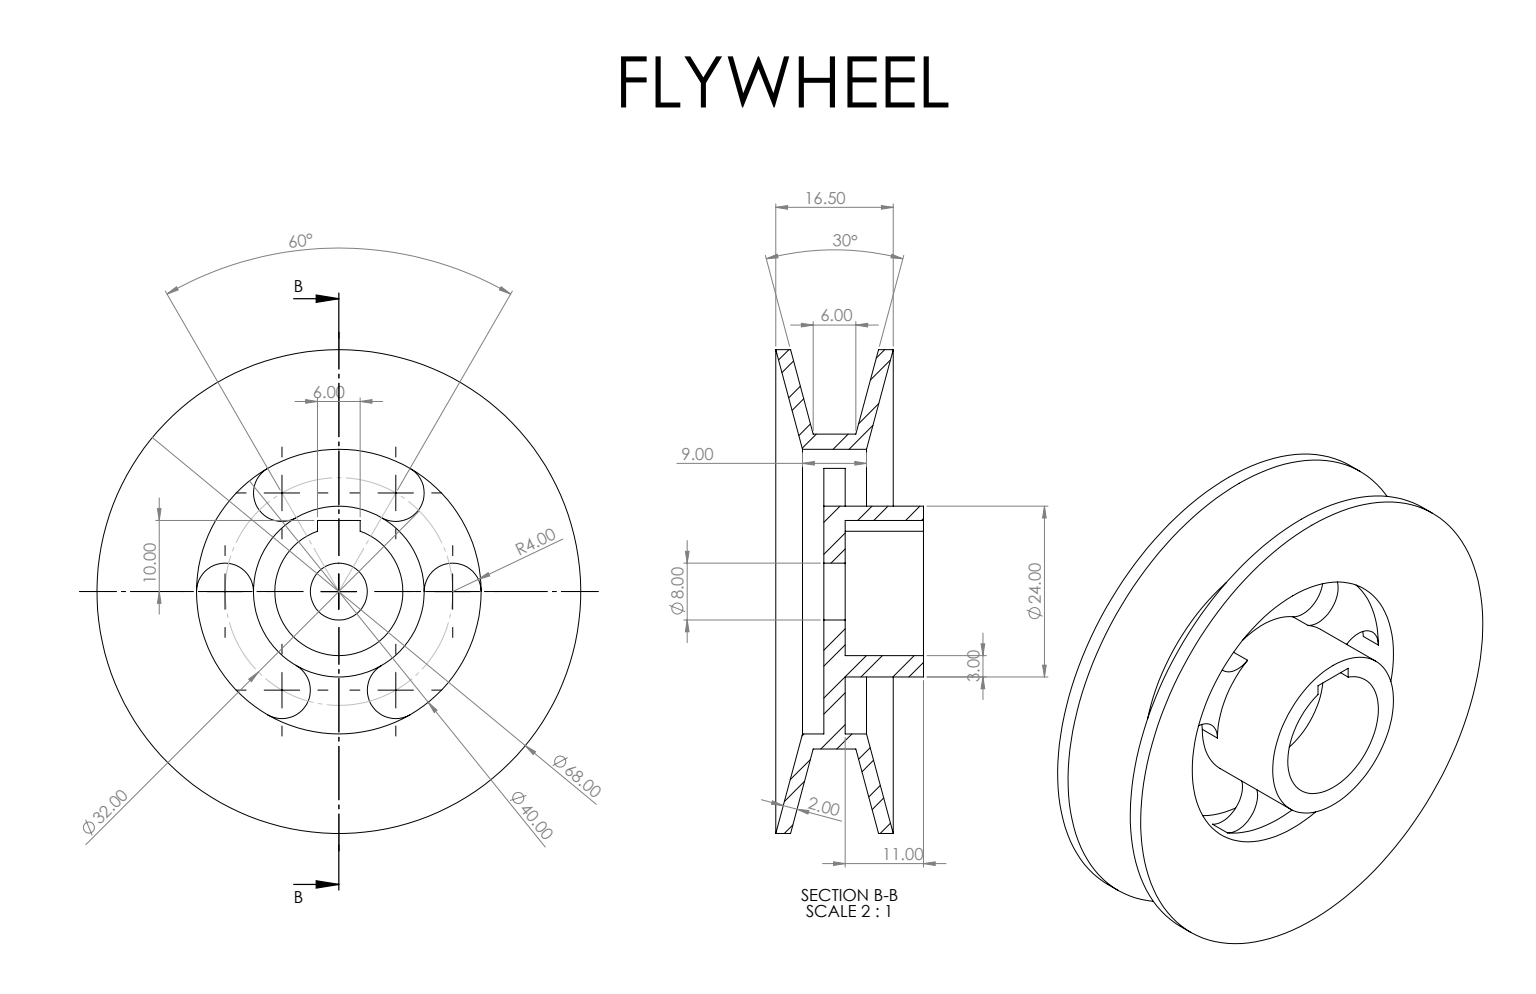
ISO-10303-21;
HEADER;
FILE_DESCRIPTION (('STEP AP214'),
    '1' );
FILE_NAME ('FLYWHEEL.step',
    '2026-10-24T00:51:42',
    ( '' ),
    ( '' ),
    'SwSTEP 2.0',
    'SolidWorks 2025',
    '' );
FILE_SCHEMA (( 'AUTOMOTIVE_DESIGN' ));
ENDSEC;

DATA;
#1=DIRECTION ( 'NONE',  ( 1.296372316667914327E-16, 1.000000000000000000, -0.000000000000000000 ) ) ;
#7=VERTEX_POINT ( 'NONE', #19816 ) ;
#14=LINE ( 'NONE', #10421, #6182 ) ;
#34=ORIENTED_EDGE ( 'NONE', *, *, #17370, .T. ) ;
#40=ORIENTED_EDGE ( 'NONE', *, *, #1892, .T. ) ;
#122=CARTESIAN_POINT ( 'NONE',  ( 4.000000000000007105, 28.19616000222403684, 4.898587196589412829E-16 ) ) ;
#157=DIRECTION ( 'NONE',  ( 0.000000000000000000, 0.000000000000000000, 1.000000000000000000 ) ) ;
#180=( LENGTH_UNIT ( ) NAMED_UNIT ( * ) SI_UNIT ( .MILLI., .METRE. ) );
#212=EDGE_LOOP ( 'NONE', ( #4099, #12246, #12145, #6281 ) ) ;
#220=AXIS2_PLACEMENT_3D ( 'NONE', #14083, #12166, #15923 ) ;
#229=ORIENTED_EDGE ( 'NONE', *, *, #280, .F. ) ;
#235=CARTESIAN_POINT ( 'NONE',  ( 34.00000000000000000, -8.251288694035739724, 4.163799117101000559E-15 ) ) ;
#250=( NAMED_UNIT ( * ) SI_UNIT ( $, .STERADIAN. ) SOLID_ANGLE_UNIT ( ) );
#252=ORIENTED_EDGE ( 'NONE', *, *, #20268, .F. ) ;
#272=VECTOR ( 'NONE', #9542, 1000.000000000000000 ) ;
#273=VECTOR ( 'NONE', #6613, 1000.000000000000000 ) ;
#280=EDGE_CURVE ( 'NONE', #4403, #3845, #2016, .T. ) ;
#286=DIRECTION ( 'NONE',  ( 1.000000000000000000, -1.084202172485504927E-16, 0.000000000000000000 ) ) ;
#298=DIRECTION ( 'NONE',  ( -1.000000000000000000, 0.000000000000000000, 0.000000000000000000 ) ) ;
#301=AXIS2_PLACEMENT_3D ( 'NONE', #19951, #21671, #11581 ) ;
#316=AXIS2_PLACEMENT_3D ( 'NONE', #15240, #12961, #19969 ) ;
#342=DIRECTION ( 'NONE',  ( -1.000000000000000000, 0.000000000000000000, 0.000000000000000000 ) ) ;
#354=DIRECTION ( 'NONE',  ( 1.296372316667914327E-16, 1.000000000000000000, -0.000000000000000000 ) ) ;
#379=CARTESIAN_POINT ( 'NONE',  ( -13.85640646055084702, -1.500000000000011768, 7.999999999999705125 ) ) ;
#395=EDGE_LOOP ( 'NONE', ( #16035, #6473, #11617, #1674 ) ) ;
#397=EDGE_CURVE ( 'NONE', #22398, #3259, #6731, .T. ) ;
#414=CIRCLE ( 'NONE', #13204, 4.000000000000000000 ) ;
#421=PLANE ( 'NONE',  #17700 ) ;
#422=CARTESIAN_POINT ( 'NONE',  ( 34.00000000000000000, 8.251288694035739724, 4.163799117100999770E-15 ) ) ;
#432=ORIENTED_EDGE ( 'NONE', *, *, #17613, .T. ) ;
#435=DIRECTION ( 'NONE',  ( -1.000000000000000000, 1.371829164384562918E-16, 0.000000000000000000 ) ) ;
#439=FACE_OUTER_BOUND ( 'NONE', #4503, .T. ) ;
#457=DIRECTION ( 'NONE',  ( 1.296372316667914327E-16, 1.000000000000000000, -0.000000000000000000 ) ) ;
#480=LINE ( 'NONE', #7251, #20898 ) ;
#494=CARTESIAN_POINT ( 'NONE',  ( 3.849727973822421485E-15, 1.499999999999994449, 0.000000000000000000 ) ) ;
#501=EDGE_CURVE ( 'NONE', #11241, #8065, #19539, .T. ) ;
#512=VECTOR ( 'NONE', #9586, 1000.000000000000000 ) ;
#517=DIRECTION ( 'NONE',  ( 1.296372316667914327E-16, 1.000000000000000000, -0.000000000000000000 ) ) ;
#518=VECTOR ( 'NONE', #17062, 1000.000000000000000 ) ;
#522=DIRECTION ( 'NONE',  ( 1.296372316667914327E-16, 1.000000000000000000, -0.000000000000000000 ) ) ;
#549=EDGE_CURVE ( 'NONE', #21392, #4403, #13704, .T. ) ;
#562=AXIS2_PLACEMENT_3D ( 'NONE', #8192, #22408, #11628 ) ;
#569=CARTESIAN_POINT ( 'NONE',  ( -13.85640646055084702, -1.500000000000011768, 11.99999999999970335 ) ) ;
#570=CIRCLE ( 'NONE', #3154, 19.99999999999999289 ) ;
#577=AXIS2_PLACEMENT_3D ( 'NONE', #19256, #1, #8819 ) ;
#598=( LENGTH_UNIT ( ) NAMED_UNIT ( * ) SI_UNIT ( .MILLI., .METRE. ) );
#610=DIRECTION ( 'NONE',  ( 1.000000000000000000, -1.301042606982605814E-16, 0.000000000000000000 ) ) ;
#621=EDGE_CURVE ( 'NONE', #21949, #5947, #10354, .T. ) ;
#626=VERTEX_POINT ( 'NONE', #3731 ) ;
#627=ORIENTED_EDGE ( 'NONE', *, *, #19282, .F. ) ;
#644=CARTESIAN_POINT ( 'NONE',  ( -22.12933039895921183, -2.999999999999992895, 0.000000000000000000 ) ) ;
#651=VERTEX_POINT ( 'NONE', #17468 ) ;
#656=AXIS2_PLACEMENT_3D ( 'NONE', #1334, #18751, #13229 ) ;
#659=CARTESIAN_POINT ( 'NONE',  ( 4.000000000000003553, -1.500000000000015099, 0.000000000000000000 ) ) ;
#669=CIRCLE ( 'NONE', #11643, 22.12933039895921539 ) ;
#676=ORIENTED_EDGE ( 'NONE', *, *, #4878, .T. ) ;
#694=DIRECTION ( 'NONE',  ( 1.296372316667914327E-16, 1.000000000000000000, -0.000000000000000000 ) ) ;
#780=CARTESIAN_POINT ( 'NONE',  ( -17.32050807568873196, -1.500000000000011768, 9.999999999999772626 ) ) ;
#782=FACE_OUTER_BOUND ( 'NONE', #19177, .T. ) ;
#793=DIRECTION ( 'NONE',  ( 1.296372316667914327E-16, 1.000000000000000000, -0.000000000000000000 ) ) ;
#881=FACE_BOUND ( 'NONE', #13282, .T. ) ;
#888=CARTESIAN_POINT ( 'NONE',  ( 34.00000000000000711, 28.19616000222403329, 4.163799117101000559E-15 ) ) ;
#902=CARTESIAN_POINT ( 'NONE',  ( 13.85640646055130709, -1.500000000000015099, -4.000000000000099476 ) ) ;
#918=DIRECTION ( 'NONE',  ( -1.000000000000000000, 0.000000000000000000, 0.000000000000000000 ) ) ;
#925=CYLINDRICAL_SURFACE ( 'NONE', #17707, 4.000000000000000000 ) ;
#931=CIRCLE ( 'NONE', #17391, 9.000000000000000000 ) ;
#946=ORIENTED_EDGE ( 'NONE', *, *, #15805, .F. ) ;
#970=VECTOR ( 'NONE', #5351, 1000.000000000000000 ) ;
#988=CARTESIAN_POINT ( 'NONE',  ( 1.734786545154649763E-13, 1.500000000000004885, -16.00000000000029488 ) ) ;
#1012=EDGE_CURVE ( 'NONE', #17260, #11580, #15474, .T. ) ;
#1095=ORIENTED_EDGE ( 'NONE', *, *, #6767, .T. ) ;
#1099=ORIENTED_EDGE ( 'NONE', *, *, #9484, .F. ) ;
#1215=VECTOR ( 'NONE', #22012, 1000.000000000000000 ) ;
#1276=CARTESIAN_POINT ( 'NONE',  ( -19.99999999999998934, 4.500000000000009770, 0.000000000000000000 ) ) ;
#1326=AXIS2_PLACEMENT_3D ( 'NONE', #12628, #3503, #21247 ) ;
#1334=CARTESIAN_POINT ( 'NONE',  ( 7.310544252644470693E-15, 28.19616000222403684, 0.000000000000000000 ) ) ;
#1341=CARTESIAN_POINT ( 'NONE',  ( -10.00000000000000000, 1.499999999999997780, 3.000000000000000000 ) ) ;
#1373=VECTOR ( 'NONE', #12449, 1000.000000000000000 ) ;
#1375=ORIENTED_EDGE ( 'NONE', *, *, #8971, .T. ) ;
#1384=CIRCLE ( 'NONE', #21527, 3.999999999999996447 ) ;
#1398=DIRECTION ( 'NONE',  ( 0.000000000000000000, 0.000000000000000000, 1.000000000000000000 ) ) ;
#1399=APPLICATION_CONTEXT ( 'automotive_design' ) ;
#1406=ORIENTED_EDGE ( 'NONE', *, *, #8971, .F. ) ;
#1427=ORIENTED_EDGE ( 'NONE', *, *, #4182, .T. ) ;
#1436=CARTESIAN_POINT ( 'NONE',  ( 20.00000000000000000, 28.19616000222403329, 2.449293598294705724E-15 ) ) ;
#1444=( GEOMETRIC_REPRESENTATION_CONTEXT ( 3 ) GLOBAL_UNCERTAINTY_ASSIGNED_CONTEXT ( ( #13302 ) ) GLOBAL_UNIT_ASSIGNED_CONTEXT ( ( #598, #9306, #250 ) ) REPRESENTATION_CONTEXT ( 'NONE', 'WORKASPACE' ) );
#1469=DIRECTION ( 'NONE',  ( 1.296372316667914327E-16, 1.000000000000000000, -0.000000000000000000 ) ) ;
#1505=EDGE_CURVE ( 'NONE', #15515, #14562, #11061, .T. ) ;
#1506=FACE_BOUND ( 'NONE', #395, .T. ) ;
#1516=ORIENTED_EDGE ( 'NONE', *, *, #3101, .T. ) ;
#1526=DIRECTION ( 'NONE',  ( -1.000000000000000000, 1.927470528863119049E-16, 0.000000000000000000 ) ) ;
#1552=ORIENTED_EDGE ( 'NONE', *, *, #2402, .F. ) ;
#1570=ORIENTED_EDGE ( 'NONE', *, *, #10768, .F. ) ;
#1595=FACE_OUTER_BOUND ( 'NONE', #17651, .T. ) ;
#1624=CARTESIAN_POINT ( 'NONE',  ( 3.849727973822421485E-15, 1.499999999999997780, 0.000000000000000000 ) ) ;
#1638=DIRECTION ( 'NONE',  ( -1.000000000000000000, 1.734723475976807834E-16, 0.000000000000000000 ) ) ;
#1642=EDGE_CURVE ( 'NONE', #7946, #651, #17286, .T. ) ;
#1648=CARTESIAN_POINT ( 'NONE',  ( 0.000000000000000000, 0.000000000000000000, 0.000000000000000000 ) ) ;
#1649=ORIENTED_EDGE ( 'NONE', *, *, #7636, .F. ) ;
#1650=DIRECTION ( 'NONE',  ( 1.296372316667914327E-16, 1.000000000000000000, -0.000000000000000000 ) ) ;
#1658=ORIENTED_EDGE ( 'NONE', *, *, #14495, .T. ) ;
#1661=EDGE_LOOP ( 'NONE', ( #6020, #16109, #16262, #15546 ) ) ;
#1663=AXIS2_PLACEMENT_3D ( 'NONE', #9499, #12798, #435 ) ;
#1664=CARTESIAN_POINT ( 'NONE',  ( -34.00000000000000000, -6.180736333215561373, 4.163799117101000559E-15 ) ) ;
#1674=ORIENTED_EDGE ( 'NONE', *, *, #1642, .T. ) ;
#1682=VECTOR ( 'NONE', #1745, 1000.000000000000000 ) ;
#1684=AXIS2_PLACEMENT_3D ( 'NONE', #17713, #14492, #2138 ) ;
#1696=AXIS2_PLACEMENT_3D ( 'NONE', #22355, #2878, #22124 ) ;
#1713=FACE_OUTER_BOUND ( 'NONE', #5783, .T. ) ;
#1735=CARTESIAN_POINT ( 'NONE',  ( 22.12933039895921894, 3.000000000000003109, 3.436930240568481542E-15 ) ) ;
#1745=DIRECTION ( 'NONE',  ( 1.296372316667914327E-16, 1.000000000000000000, -0.000000000000000000 ) ) ;
#1747=ORIENTED_EDGE ( 'NONE', *, *, #6797, .T. ) ;
#1756=FACE_OUTER_BOUND ( 'NONE', #13620, .T. ) ;
#1775=ORIENTED_EDGE ( 'NONE', *, *, #13470, .T. ) ;
#1788=CARTESIAN_POINT ( 'NONE',  ( -2.467804172277818612E-14, 1.500000000000002887, 11.99999999999966960 ) ) ;
#1797=DIRECTION ( 'NONE',  ( 1.296372316667914327E-16, 1.000000000000000000, -0.000000000000000000 ) ) ;
#1808=CARTESIAN_POINT ( 'NONE',  ( -22.12933039895921183, 3.000000000000009326, 0.000000000000000000 ) ) ;
#1892=EDGE_CURVE ( 'NONE', #8190, #7904, #20239, .T. ) ;
#1895=AXIS2_PLACEMENT_3D ( 'NONE', #17411, #3457, #6656 ) ;
#1898=ORIENTED_EDGE ( 'NONE', *, *, #11064, .F. ) ;
#1918=ORIENTED_EDGE ( 'NONE', *, *, #10579, .T. ) ;
#1985=VERTEX_POINT ( 'NONE', #12497 ) ;
#2016=CIRCLE ( 'NONE', #19183, 19.99999999999999289 ) ;
#2024=CARTESIAN_POINT ( 'NONE',  ( -10.39230484541309174, -1.500000000000011768, 5.999999999999708677 ) ) ;
#2027=ORIENTED_EDGE ( 'NONE', *, *, #12241, .F. ) ;
#2044=ORIENTED_EDGE ( 'NONE', *, *, #10253, .T. ) ;
#2061=DIRECTION ( 'NONE',  ( 0.000000000000000000, 0.000000000000000000, 1.000000000000000000 ) ) ;
#2132=DIRECTION ( 'NONE',  ( -0.000000000000000000, 1.000000000000000000, -0.000000000000000000 ) ) ;
#2137=CYLINDRICAL_SURFACE ( 'NONE', #9464, 8.999999999999998224 ) ;
#2138=DIRECTION ( 'NONE',  ( -1.000000000000000000, 1.084202172485504434E-16, 0.000000000000000000 ) ) ;
#2160=CARTESIAN_POINT ( 'NONE',  ( -10.00000000000000000, 1.499999999999997780, 3.000000000000000000 ) ) ;
#2189=ADVANCED_FACE ( 'NONE', ( #6551 ), #19147, .T. ) ;
#2257=EDGE_LOOP ( 'NONE', ( #1570, #15899 ) ) ;
#2264=DIRECTION ( 'NONE',  ( 1.296372316667914327E-16, 1.000000000000000000, -0.000000000000000000 ) ) ;
#2296=EDGE_CURVE ( 'NONE', #10675, #16483, #414, .T. ) ;
#2304=VERTEX_POINT ( 'NONE', #569 ) ;
#2307=DIRECTION ( 'NONE',  ( 1.296372316667914327E-16, 1.000000000000000000, -0.000000000000000000 ) ) ;
#2362=DIRECTION ( 'NONE',  ( -1.000000000000000000, 1.371829164384562918E-16, 0.000000000000000000 ) ) ;
#2369=AXIS2_PLACEMENT_3D ( 'NONE', #22218, #1469, #20718 ) ;
#2376=CARTESIAN_POINT ( 'NONE',  ( 9.000000000000005329, 12.49999999999999467, 0.000000000000000000 ) ) ;
#2377=CLOSED_SHELL ( 'NONE', ( #15840, #2588, #18828, #3195, #14125, #19318, #13827, #6682, #21945, #10747, #17338, #14273, #22672, #14010, #8312, #12983, #9918, #6676, #7246, #21227, #12866, #3900, #16028, #2189, #18705, #11982, #13364, #12111, #21806, #17586, #11435, #17237, #8288, #21448, #10491, #16012, #20701, #9854 ) ) ;
#2380=EDGE_CURVE ( 'NONE', #8634, #18457, #2887, .T. ) ;
#2402=EDGE_CURVE ( 'NONE', #12588, #11670, #15669, .T. ) ;
#2415=ORIENTED_EDGE ( 'NONE', *, *, #1505, .T. ) ;
#2424=CARTESIAN_POINT ( 'NONE',  ( 12.00000000000000355, 1.499999999999996447, 1.469576158976823947E-15 ) ) ;
#2449=ORIENTED_EDGE ( 'NONE', *, *, #5012, .F. ) ;
#2475=CYLINDRICAL_SURFACE ( 'NONE', #21721, 12.00000000000000000 ) ;
#2497=CARTESIAN_POINT ( 'NONE',  ( 4.044183821322609990E-15, 3.000000000000006217, 0.000000000000000000 ) ) ;
#2507=DIRECTION ( 'NONE',  ( -1.000000000000000000, 1.567804759296643123E-16, 0.000000000000000000 ) ) ;
#2511=VECTOR ( 'NONE', #20802, 1000.000000000000000 ) ;
#2514=DIRECTION ( 'NONE',  ( -1.000000000000000000, 0.000000000000000000, -0.000000000000000000 ) ) ;
#2530=ORIENTED_EDGE ( 'NONE', *, *, #6684, .T. ) ;
#2575=STYLED_ITEM('',(#22748),#18432);
#2588=ADVANCED_FACE ( 'NONE', ( #9466 ), #19884, .F. ) ;
#2610=FACE_BOUND ( 'NONE', #18350, .T. ) ;
#2630=EDGE_CURVE ( 'NONE', #3259, #22398, #13450, .T. ) ;
#2640=CARTESIAN_POINT ( 'NONE',  ( -13.85640646055084702, -25.00000000000000000, 7.999999999999705125 ) ) ;
#2659=EDGE_CURVE ( 'NONE', #6902, #13173, #9095, .T. ) ;
#2683=DIRECTION ( 'NONE',  ( -1.000000000000000000, 1.530638361156006245E-16, 0.000000000000000000 ) ) ;
#2739=CARTESIAN_POINT ( 'NONE',  ( -33.99999999999998579, 8.251288694035750382, 0.000000000000000000 ) ) ;
#2745=EDGE_CURVE ( 'NONE', #8634, #14562, #13436, .T. ) ;
#2747=CARTESIAN_POINT ( 'NONE',  ( -4.359932693009644117E-14, -1.500000000000015987, 19.99999999999999289 ) ) ;
#2803=AXIS2_PLACEMENT_3D ( 'NONE', #18547, #21883, #16594 ) ;
#2812=ORIENTED_EDGE ( 'NONE', *, *, #21989, .F. ) ;
#2821=DIRECTION ( 'NONE',  ( 1.296372316667914327E-16, 1.000000000000000000, -0.000000000000000000 ) ) ;
#2829=EDGE_CURVE ( 'NONE', #18519, #22196, #7986, .T. ) ;
#2831=ORIENTED_EDGE ( 'NONE', *, *, #18843, .T. ) ;
#2847=AXIS2_PLACEMENT_3D ( 'NONE', #3112, #11479, #18699 ) ;
#2871=DIRECTION ( 'NONE',  ( 1.296372316667914327E-16, 1.000000000000000000, -0.000000000000000000 ) ) ;
#2878=DIRECTION ( 'NONE',  ( 1.296372316667914327E-16, 1.000000000000000000, -0.000000000000000000 ) ) ;
#2887=CIRCLE ( 'NONE', #3984, 22.12933039895921539 ) ;
#2903=FACE_OUTER_BOUND ( 'NONE', #3500, .T. ) ;
#2924=AXIS2_PLACEMENT_3D ( 'NONE', #12514, #12753, #3836 ) ;
#2961=LINE ( 'NONE', #7881, #22187 ) ;
#3024=CYLINDRICAL_SURFACE ( 'NONE', #17665, 34.00000000000000000 ) ;
#3101=EDGE_CURVE ( 'NONE', #5844, #9303, #19375, .T. ) ;
#3103=ORIENTED_EDGE ( 'NONE', *, *, #397, .F. ) ;
#3112=CARTESIAN_POINT ( 'NONE',  ( 3.071904583821672593E-15, -4.500000000000010658, 0.000000000000000000 ) ) ;
#3115=CARTESIAN_POINT ( 'NONE',  ( -22.12933039895921183, 3.000000000000009326, 0.000000000000000000 ) ) ;
#3154=AXIS2_PLACEMENT_3D ( 'NONE', #8531, #8978, #7380 ) ;
#3161=AXIS2_PLACEMENT_3D ( 'NONE', #22565, #17265, #13584 ) ;
#3163=EDGE_CURVE ( 'NONE', #17046, #6470, #17144, .T. ) ;
#3174=AXIS2_PLACEMENT_3D ( 'NONE', #3756, #12999, #4437 ) ;
#3195=ADVANCED_FACE ( 'NONE', ( #2903 ), #9110, .F. ) ;
#3233=FACE_OUTER_BOUND ( 'NONE', #11673, .T. ) ;
#3254=CARTESIAN_POINT ( 'NONE',  ( 5.275737522157127195E-15, 12.49999999999999645, 0.000000000000000000 ) ) ;
#3259=VERTEX_POINT ( 'NONE', #3115 ) ;
#3291=ORIENTED_EDGE ( 'NONE', *, *, #10893, .F. ) ;
#3292=CARTESIAN_POINT ( 'NONE',  ( 2.854018578421813982E-15, -6.180736333215565814, 0.000000000000000000 ) ) ;
#3303=LINE ( 'NONE', #1341, #273 ) ;
#3314=CIRCLE ( 'NONE', #14983, 19.99999999999999289 ) ;
#3317=EDGE_CURVE ( 'NONE', #4351, #21949, #14, .T. ) ;
#3334=CARTESIAN_POINT ( 'NONE',  ( 12.00000000000000711, 28.19616000222403684, 1.469576158976823947E-15 ) ) ;
#3355=CARTESIAN_POINT ( 'NONE',  ( -10.39230484541300825, -1.500000000000011768, -6.000000000000442313 ) ) ;
#3362=ORIENTED_EDGE ( 'NONE', *, *, #549, .F. ) ;
#3363=CARTESIAN_POINT ( 'NONE',  ( 6.383438919230843859E-14, -25.00000000000000000, -20.00000000000029488 ) ) ;
#3367=CARTESIAN_POINT ( 'NONE',  ( 7.310544252644470693E-15, 28.19616000222403684, 0.000000000000000000 ) ) ;
#3401=EDGE_CURVE ( 'NONE', #7, #1985, #4720, .T. ) ;
#3402=CARTESIAN_POINT ( 'NONE',  ( -8.485281374238564212, 12.49999999999999822, -3.000000000000000000 ) ) ;
#3407=ORIENTED_EDGE ( 'NONE', *, *, #12251, .F. ) ;
#3446=PLANE ( 'NONE',  #9367 ) ;
#3457=DIRECTION ( 'NONE',  ( 1.296372316667914327E-16, 1.000000000000000000, -0.000000000000000000 ) ) ;
#3467=DIRECTION ( 'NONE',  ( 1.296372316667914327E-16, 1.000000000000000000, -0.000000000000000000 ) ) ;
#3475=ORIENTED_EDGE ( 'NONE', *, *, #2296, .F. ) ;
#3500=EDGE_LOOP ( 'NONE', ( #2831, #8629, #10943, #13779 ) ) ;
#3503=DIRECTION ( 'NONE',  ( 1.296372316667914327E-16, 1.000000000000000000, -0.000000000000000000 ) ) ;
#3511=EDGE_LOOP ( 'NONE', ( #18181, #22428, #18359, #11116 ) ) ;
#3519=DIRECTION ( 'NONE',  ( -1.000000000000000000, 1.264902534566421922E-16, 0.000000000000000000 ) ) ;
#3541=ORIENTED_EDGE ( 'NONE', *, *, #7207, .F. ) ;
#3550=CARTESIAN_POINT ( 'NONE',  ( 7.310544252644470693E-15, 28.19616000222403684, 0.000000000000000000 ) ) ;
#3555=AXIS2_PLACEMENT_3D ( 'NONE', #21855, #6153, #16567 ) ;
#3565=EDGE_CURVE ( 'NONE', #20227, #17027, #10702, .T. ) ;
#3573=VECTOR ( 'NONE', #18015, 1000.000000000000000 ) ;
#3583=LINE ( 'NONE', #7883, #7896 ) ;
#3612=DIRECTION ( 'NONE',  ( 1.296372316667914327E-16, 1.000000000000000000, -0.000000000000000000 ) ) ;
#3616=ORIENTED_EDGE ( 'NONE', *, *, #3163, .F. ) ;
#3635=VERTEX_POINT ( 'NONE', #11450 ) ;
#3669=ORIENTED_EDGE ( 'NONE', *, *, #10893, .T. ) ;
#3671=DIRECTION ( 'NONE',  ( 1.296372316667914327E-16, 1.000000000000000000, -0.000000000000000000 ) ) ;
#3731=CARTESIAN_POINT ( 'NONE',  ( 13.85640646055130709, 1.500000000000004885, -4.000000000000099476 ) ) ;
#3756=CARTESIAN_POINT ( 'NONE',  ( 3.849727973822421485E-15, 1.499999999999997780, 0.000000000000000000 ) ) ;
#3771=DIRECTION ( 'NONE',  ( 0.9659258262890680902, -0.2588190451025210170, 0.000000000000000000 ) ) ;
#3778=CARTESIAN_POINT ( 'NONE',  ( 12.00000000000000355, 1.500000000000003553, 0.000000000000000000 ) ) ;
#3780=VECTOR ( 'NONE', #5970, 1000.000000000000000 ) ;
#3825=CARTESIAN_POINT ( 'NONE',  ( 10.39230484541348432, 1.500000000000003109, -6.000000000000073719 ) ) ;
#3827=LINE ( 'NONE', #3942, #3573 ) ;
#3836=DIRECTION ( 'NONE',  ( -1.000000000000000000, 1.301042606982605814E-16, 0.000000000000000000 ) ) ;
#3845=VERTEX_POINT ( 'NONE', #4000 ) ;
#3847=EDGE_LOOP ( 'NONE', ( #20703, #21022, #16887, #11706 ) ) ;
#3855=CIRCLE ( 'NONE', #9702, 11.99999999999985256 ) ;
#3859=DIRECTION ( 'NONE',  ( -1.000000000000000000, 1.084202172485504927E-16, 0.000000000000000000 ) ) ;
#3889=ORIENTED_EDGE ( 'NONE', *, *, #2659, .F. ) ;
#3891=CARTESIAN_POINT ( 'NONE',  ( -10.00000000000000000, -4.824555320336763486, -3.000000000000000000 ) ) ;
#3900=ADVANCED_FACE ( 'NONE', ( #21293 ), #8809, .T. ) ;
#3919=DIRECTION ( 'NONE',  ( -1.296372316667914327E-16, -1.000000000000000000, 0.000000000000000000 ) ) ;
#3942=CARTESIAN_POINT ( 'NONE',  ( -8.485281374238560659, 28.19616000222403684, -3.000000000000000000 ) ) ;
#3964=ORIENTED_EDGE ( 'NONE', *, *, #10073, .F. ) ;
#3984=AXIS2_PLACEMENT_3D ( 'NONE', #12211, #19213, #19095 ) ;
#3994=DIRECTION ( 'NONE',  ( -1.000000000000000000, 1.371829164384562918E-16, 0.000000000000000000 ) ) ;
#4000=CARTESIAN_POINT ( 'NONE',  ( 17.32050807568880657, -1.500000000000015987, -9.999999999999934275 ) ) ;
#4004=CARTESIAN_POINT ( 'NONE',  ( 20.00000000000000000, 28.19616000222403329, 2.449293598294705724E-15 ) ) ;
#4014=CARTESIAN_POINT ( 'NONE',  ( -9.999999999999998224, 12.49999999999999822, 3.000000000000000000 ) ) ;
#4044=VERTEX_POINT ( 'NONE', #4106 ) ;
#4053=CARTESIAN_POINT ( 'NONE',  ( -8.485281374238564212, 1.499999999999997558, -3.000000000000000000 ) ) ;
#4099=ORIENTED_EDGE ( 'NONE', *, *, #21744, .F. ) ;
#4106=CARTESIAN_POINT ( 'NONE',  ( -8.485281374238564212, 12.49999999999999822, 3.000000000000000000 ) ) ;
#4147=DIRECTION ( 'NONE',  ( 1.296372316667914327E-16, 1.000000000000000000, -0.000000000000000000 ) ) ;
#4182=EDGE_CURVE ( 'NONE', #5980, #4044, #8889, .T. ) ;
#4192=CONICAL_SURFACE ( 'NONE', #6735, 22.12933039895921539, 1.308996938995746095 ) ;
#4230=LINE ( 'NONE', #2739, #17492 ) ;
#4231=AXIS2_PLACEMENT_3D ( 'NONE', #7568, #457, #918 ) ;
#4299=EDGE_CURVE ( 'NONE', #14562, #15515, #14533, .T. ) ;
#4332=CARTESIAN_POINT ( 'NONE',  ( 0.000000000000000000, -25.00000000000000000, 11.99999999999985256 ) ) ;
#4351=VERTEX_POINT ( 'NONE', #4053 ) ;
#4354=DIRECTION ( 'NONE',  ( 1.296372316667914327E-16, 1.000000000000000000, -0.000000000000000000 ) ) ;
#4380=PRODUCT_DEFINITION_SHAPE ( 'NONE', 'NONE',  #17947 ) ;
#4392=CARTESIAN_POINT ( 'NONE',  ( 3.071904583821672593E-15, -4.500000000000010658, 0.000000000000000000 ) ) ;
#4403=VERTEX_POINT ( 'NONE', #18462 ) ;
#4407=UNCERTAINTY_MEASURE_WITH_UNIT (LENGTH_MEASURE( 1.000000000000000082E-05 ), #180, 'distance_accuracy_value', 'NONE');
#4437=DIRECTION ( 'NONE',  ( -1.000000000000000000, 1.264902534566421922E-16, 0.000000000000000000 ) ) ;
#4446=DIRECTION ( 'NONE',  ( -1.000000000000000000, 1.084202172485504434E-16, 0.000000000000000000 ) ) ;
#4475=DIRECTION ( 'NONE',  ( -0.000000000000000000, 1.000000000000000000, -0.000000000000000000 ) ) ;
#4503=EDGE_LOOP ( 'NONE', ( #16138, #13930, #14702, #3407 ) ) ;
#4540=ORIENTED_EDGE ( 'NONE', *, *, #11064, .T. ) ;
#4548=AXIS2_PLACEMENT_3D ( 'NONE', #988, #13222, #16801 ) ;
#4580=EDGE_CURVE ( 'NONE', #5486, #5841, #20871, .T. ) ;
#4592=EDGE_CURVE ( 'NONE', #17027, #20227, #5906, .T. ) ;
#4599=CIRCLE ( 'NONE', #562, 3.999999999999996447 ) ;
#4614=CARTESIAN_POINT ( 'NONE',  ( 0.000000000000000000, 1.500000000000015099, 19.99999999999999645 ) ) ;
#4622=EDGE_CURVE ( 'NONE', #8683, #5161, #12467, .T. ) ;
#4633=AXIS2_PLACEMENT_3D ( 'NONE', #13899, #15504, #17117 ) ;
#4654=CONICAL_SURFACE ( 'NONE', #7559, 19.99999999999999289, 1.308996938995746984 ) ;
#4665=EDGE_LOOP ( 'NONE', ( #8035, #2027, #11749, #12833 ) ) ;
#4676=ORIENTED_EDGE ( 'NONE', *, *, #3401, .F. ) ;
#4696=EDGE_LOOP ( 'NONE', ( #14995, #20897, #432, #14474 ) ) ;
#4704=AXIS2_PLACEMENT_3D ( 'NONE', #8446, #5352, #8891 ) ;
#4717=ORIENTED_EDGE ( 'NONE', *, *, #621, .F. ) ;
#4720=CIRCLE ( 'NONE', #18620, 33.99999999999999289 ) ;
#4741=EDGE_LOOP ( 'NONE', ( #1552, #1747, #1516, #16833, #19996 ) ) ;
#4798=FACE_OUTER_BOUND ( 'NONE', #17306, .T. ) ;
#4799=FACE_BOUND ( 'NONE', #2257, .T. ) ;
#4812=CARTESIAN_POINT ( 'NONE',  ( -13.85640646055084702, 1.500000000000008216, 11.99999999999970335 ) ) ;
#4831=ORIENTED_EDGE ( 'NONE', *, *, #10006, .T. ) ;
#4878=EDGE_CURVE ( 'NONE', #18308, #22383, #7725, .T. ) ;
#4914=VECTOR ( 'NONE', #6786, 1000.000000000000000 ) ;
#4943=CARTESIAN_POINT ( 'NONE',  ( -13.85640646055073333, -1.500000000000011768, -8.000000000000493827 ) ) ;
#4964=DIRECTION ( 'NONE',  ( 1.296372316667914327E-16, 1.000000000000000000, -0.000000000000000000 ) ) ;
#5012=EDGE_CURVE ( 'NONE', #8634, #22398, #15947, .T. ) ;
#5014=CARTESIAN_POINT ( 'NONE',  ( 0.000000000000000000, -1.500000000000015099, 0.000000000000000000 ) ) ;
#5029=AXIS2_PLACEMENT_3D ( 'NONE', #379, #9319, #7372 ) ;
#5064=VECTOR ( 'NONE', #13684, 1000.000000000000000 ) ;
#5076=CARTESIAN_POINT ( 'NONE',  ( 1.734786545154649763E-13, -25.00000000000000000, -16.00000000000029488 ) ) ;
#5085=AXIS2_PLACEMENT_3D ( 'NONE', #21491, #2132, #11287 ) ;
#5106=DIRECTION ( 'NONE',  ( -1.000000000000000000, 1.301042606982605814E-16, 0.000000000000000000 ) ) ;
#5114=EDGE_CURVE ( 'NONE', #21949, #3635, #5764, .T. ) ;
#5161=VERTEX_POINT ( 'NONE', #12847 ) ;
#5165=EDGE_CURVE ( 'NONE', #6470, #8079, #16069, .T. ) ;
#5175=DIRECTION ( 'NONE',  ( -0.000000000000000000, 1.000000000000000000, -0.000000000000000000 ) ) ;
#5201=DIRECTION ( 'NONE',  ( -1.000000000000000000, 1.264902534566421922E-16, 0.000000000000000000 ) ) ;
#5214=ORIENTED_EDGE ( 'NONE', *, *, #14943, .F. ) ;
#5224=VERTEX_POINT ( 'NONE', #3825 ) ;
#5238=DIRECTION ( 'NONE',  ( 1.296372316667914327E-16, 1.000000000000000000, -0.000000000000000000 ) ) ;
#5271=FACE_OUTER_BOUND ( 'NONE', #8780, .T. ) ;
#5302=VECTOR ( 'NONE', #18204, 1000.000000000000000 ) ;
#5348=VECTOR ( 'NONE', #10037, 1000.000000000000000 ) ;
#5351=DIRECTION ( 'NONE',  ( 1.000000000000000000, 0.000000000000000000, 0.000000000000000000 ) ) ;
#5352=DIRECTION ( 'NONE',  ( -1.000000000000000000, 1.296372316667914327E-16, 0.000000000000000000 ) ) ;
#5377=DIRECTION ( 'NONE',  ( 1.296372316667914327E-16, 1.000000000000000000, -0.000000000000000000 ) ) ;
#5390=CYLINDRICAL_SURFACE ( 'NONE', #13149, 4.000000000000000000 ) ;
#5450=EDGE_CURVE ( 'NONE', #9647, #9303, #12155, .T. ) ;
#5452=AXIS2_PLACEMENT_3D ( 'NONE', #11104, #694, #21657 ) ;
#5486=VERTEX_POINT ( 'NONE', #15358 ) ;
#5504=DIRECTION ( 'NONE',  ( -1.000000000000000000, 1.530638361156006492E-16, 0.000000000000000000 ) ) ;
#5506=EDGE_LOOP ( 'NONE', ( #2812, #6535, #8458, #6349 ) ) ;
#5514=ORIENTED_EDGE ( 'NONE', *, *, #4878, .F. ) ;
#5595=CONICAL_SURFACE ( 'NONE', #8535, 33.99999999999999289, 1.308996938995745873 ) ;
#5605=DIRECTION ( 'NONE',  ( -0.000000000000000000, 1.000000000000000000, -0.000000000000000000 ) ) ;
#5620=CARTESIAN_POINT ( 'NONE',  ( -13.85640646055073333, 1.500000000000008216, -8.000000000000493827 ) ) ;
#5650=CARTESIAN_POINT ( 'NONE',  ( 22.12933039895921894, 3.000000000000003109, 2.710061364035962525E-15 ) ) ;
#5671=DIRECTION ( 'NONE',  ( 1.000000000000000000, -1.084202172485464991E-16, 0.000000000000000000 ) ) ;
#5672=CARTESIAN_POINT ( 'NONE',  ( -11.99999999999999289, 28.19616000222403684, 0.000000000000000000 ) ) ;
#5681=FACE_OUTER_BOUND ( 'NONE', #10634, .T. ) ;
#5685=DIRECTION ( 'NONE',  ( -1.000000000000000000, 1.301042606982605814E-16, 0.000000000000000000 ) ) ;
#5753=AXIS2_PLACEMENT_3D ( 'NONE', #1624, #8832, #17084 ) ;
#5764=LINE ( 'NONE', #11253, #20042 ) ;
#5774=AXIS2_PLACEMENT_3D ( 'NONE', #9311, #14445, #21455 ) ;
#5783=EDGE_LOOP ( 'NONE', ( #8667, #15668, #3669, #3541 ) ) ;
#5787=ORIENTED_EDGE ( 'NONE', *, *, #10657, .T. ) ;
#5789=DIRECTION ( 'NONE',  ( -1.000000000000000000, 1.301042606982605814E-16, 0.000000000000000000 ) ) ;
#5810=CIRCLE ( 'NONE', #11664, 12.00000000000000000 ) ;
#5835=DIRECTION ( 'NONE',  ( 0.000000000000000000, 0.000000000000000000, 1.000000000000000000 ) ) ;
#5841=VERTEX_POINT ( 'NONE', #22579 ) ;
#5844=VERTEX_POINT ( 'NONE', #4812 ) ;
#5885=CARTESIAN_POINT ( 'NONE',  ( 4.456525674222657894E-15, 6.180736333215575584, 0.000000000000000000 ) ) ;
#5900=ORIENTED_EDGE ( 'NONE', *, *, #2829, .F. ) ;
#5904=CARTESIAN_POINT ( 'NONE',  ( 13.85640646055118808, 1.500000000000004885, 7.999999999999710454 ) ) ;
#5906=CIRCLE ( 'NONE', #11394, 11.99999999999999822 ) ;
#5923=ORIENTED_EDGE ( 'NONE', *, *, #280, .T. ) ;
#5941=DIRECTION ( 'NONE',  ( -1.000000000000000000, 1.020425574104004122E-16, 0.000000000000000000 ) ) ;
#5947=VERTEX_POINT ( 'NONE', #2160 ) ;
#5960=LINE ( 'NONE', #6194, #13055 ) ;
#5970=DIRECTION ( 'NONE',  ( 1.296372316667914327E-16, 1.000000000000000000, -0.000000000000000000 ) ) ;
#5974=ORIENTED_EDGE ( 'NONE', *, *, #13218, .F. ) ;
#5980=VERTEX_POINT ( 'NONE', #6385 ) ;
#5984=CARTESIAN_POINT ( 'NONE',  ( 2.854018578421813982E-15, -6.180736333215565814, 0.000000000000000000 ) ) ;
#5987=CARTESIAN_POINT ( 'NONE',  ( -13.85640646055084702, 1.500000000000008216, 7.999999999999705125 ) ) ;
#6000=DIRECTION ( 'NONE',  ( -0.000000000000000000, 1.000000000000000000, -0.000000000000000000 ) ) ;
#6020=ORIENTED_EDGE ( 'NONE', *, *, #14495, .F. ) ;
#6071=ADVANCED_BREP_SHAPE_REPRESENTATION ( '', ( #18432, #18273 ), #1444 ) ;
#6103=EDGE_LOOP ( 'NONE', ( #1898, #252, #6115, #10136 ) ) ;
#6115=ORIENTED_EDGE ( 'NONE', *, *, #19164, .T. ) ;
#6135=ORIENTED_EDGE ( 'NONE', *, *, #621, .T. ) ;
#6153=DIRECTION ( 'NONE',  ( 1.296372316667914327E-16, 1.000000000000000000, -0.000000000000000000 ) ) ;
#6165=VECTOR ( 'NONE', #21643, 1000.000000000000000 ) ;
#6182=VECTOR ( 'NONE', #19271, 1000.000000000000000 ) ;
#6191=DIRECTION ( 'NONE',  ( -1.000000000000000000, 1.445602896647339410E-16, 0.000000000000000000 ) ) ;
#6194=CARTESIAN_POINT ( 'NONE',  ( 34.00000000000000000, 28.19616000222403329, 4.163799117100999770E-15 ) ) ;
#6244=ORIENTED_EDGE ( 'NONE', *, *, #14854, .F. ) ;
#6250=DIRECTION ( 'NONE',  ( -1.000000000000000000, 1.264902534566437206E-16, 0.000000000000000000 ) ) ;
#6271=EDGE_CURVE ( 'NONE', #22398, #8190, #14582, .T. ) ;
#6281=ORIENTED_EDGE ( 'NONE', *, *, #3401, .T. ) ;
#6312=ORIENTED_EDGE ( 'NONE', *, *, #10579, .F. ) ;
#6349=ORIENTED_EDGE ( 'NONE', *, *, #3101, .F. ) ;
#6385=CARTESIAN_POINT ( 'NONE',  ( -9.999999999999998224, 12.49999999999999645, 3.000000000000000000 ) ) ;
#6438=CARTESIAN_POINT ( 'NONE',  ( 7.310544252644470693E-15, 28.19616000222403684, 0.000000000000000000 ) ) ;
#6455=CIRCLE ( 'NONE', #11584, 34.00000000000000000 ) ;
#6460=FACE_OUTER_BOUND ( 'NONE', #11533, .T. ) ;
#6470=VERTEX_POINT ( 'NONE', #2747 ) ;
#6473=ORIENTED_EDGE ( 'NONE', *, *, #15600, .F. ) ;
#6506=CARTESIAN_POINT ( 'NONE',  ( 19.99999999999999645, 4.500000000000004441, 3.306546357697853339E-15 ) ) ;
#6535=ORIENTED_EDGE ( 'NONE', *, *, #8991, .F. ) ;
#6537=DIRECTION ( 'NONE',  ( -0.000000000000000000, 1.000000000000000000, -0.000000000000000000 ) ) ;
#6551=FACE_OUTER_BOUND ( 'NONE', #8338, .T. ) ;
#6564=DIRECTION ( 'NONE',  ( -0.000000000000000000, 1.000000000000000000, -0.000000000000000000 ) ) ;
#6580=ORIENTED_EDGE ( 'NONE', *, *, #1642, .F. ) ;
#6583=ORIENTED_EDGE ( 'NONE', *, *, #14854, .T. ) ;
#6613=DIRECTION ( 'NONE',  ( 1.000000000000000000, -1.296372316667914327E-16, 0.000000000000000000 ) ) ;
#6632=AXIS2_PLACEMENT_3D ( 'NONE', #13129, #20142, #4446 ) ;
#6656=DIRECTION ( 'NONE',  ( -1.000000000000000000, 1.567804759296643123E-16, 0.000000000000000000 ) ) ;
#6663=ORIENTED_EDGE ( 'NONE', *, *, #13981, .F. ) ;
#6676=ADVANCED_FACE ( 'NONE', ( #2610, #9139 ), #421, .F. ) ;
#6682=ADVANCED_FACE ( 'NONE', ( #19690 ), #4192, .T. ) ;
#6684=EDGE_CURVE ( 'NONE', #16002, #5224, #16112, .T. ) ;
#6731=CIRCLE ( 'NONE', #8956, 22.12933039895921539 ) ;
#6735=AXIS2_PLACEMENT_3D ( 'NONE', #2497, #19568, #3994 ) ;
#6767=EDGE_CURVE ( 'NONE', #17046, #11670, #19905, .T. ) ;
#6773=CARTESIAN_POINT ( 'NONE',  ( 5.275737522157127195E-15, 12.49999999999999645, 0.000000000000000000 ) ) ;
#6780=CARTESIAN_POINT ( 'NONE',  ( -17.32050807568873196, -25.00000000000000000, 9.999999999999772626 ) ) ;
#6786=DIRECTION ( 'NONE',  ( -0.000000000000000000, 1.000000000000000000, -0.000000000000000000 ) ) ;
#6797=EDGE_CURVE ( 'NONE', #12588, #5844, #19916, .T. ) ;
#6798=AXIS2_PLACEMENT_3D ( 'NONE', #5885, #16178, #14112 ) ;
#6811=ORIENTED_EDGE ( 'NONE', *, *, #10940, .F. ) ;
#6817=VECTOR ( 'NONE', #7039, 1000.000000000000000 ) ;
#6833=CIRCLE ( 'NONE', #1696, 8.999999999999998224 ) ;
#6902=VERTEX_POINT ( 'NONE', #22422 ) ;
#6933=ORIENTED_EDGE ( 'NONE', *, *, #13188, .F. ) ;
#6943=CARTESIAN_POINT ( 'NONE',  ( 13.85640646055130709, 1.500000000000004885, -8.000000000000097700 ) ) ;
#6963=DIRECTION ( 'NONE',  ( -1.296372316667914327E-16, -1.000000000000000000, 0.000000000000000000 ) ) ;
#6965=AXIS2_PLACEMENT_3D ( 'NONE', #15797, #5605, #2061 ) ;
#7008=CARTESIAN_POINT ( 'NONE',  ( 17.32050807568869644, 1.500000000000015099, 10.00000000000013323 ) ) ;
#7021=ORIENTED_EDGE ( 'NONE', *, *, #13765, .T. ) ;
#7032=VERTEX_POINT ( 'NONE', #3402 ) ;
#7039=DIRECTION ( 'NONE',  ( 1.296372316667914327E-16, 1.000000000000000000, -0.000000000000000000 ) ) ;
#7134=DIRECTION ( 'NONE',  ( -0.9659258262890683122, -0.2588190451025209060, 1.182917971378669595E-16 ) ) ;
#7143=ORIENTED_EDGE ( 'NONE', *, *, #13244, .F. ) ;
#7201=DIRECTION ( 'NONE',  ( -0.000000000000000000, 1.000000000000000000, -0.000000000000000000 ) ) ;
#7207=EDGE_CURVE ( 'NONE', #5841, #9227, #16574, .T. ) ;
#7211=ORIENTED_EDGE ( 'NONE', *, *, #13188, .T. ) ;
#7240=EDGE_CURVE ( 'NONE', #8079, #11670, #18044, .T. ) ;
#7244=ORIENTED_EDGE ( 'NONE', *, *, #12251, .T. ) ;
#7246=ADVANCED_FACE ( 'NONE', ( #7509 ), #2475, .T. ) ;
#7251=CARTESIAN_POINT ( 'NONE',  ( -19.99999999999998934, -4.500000000000007994, 2.449293598294705724E-15 ) ) ;
#7272=DIRECTION ( 'NONE',  ( -1.000000000000000000, 1.084202172485504434E-16, 0.000000000000000000 ) ) ;
#7310=CIRCLE ( 'NONE', #20130, 4.000000000000001776 ) ;
#7321=FACE_OUTER_BOUND ( 'NONE', #7732, .T. ) ;
#7364=CARTESIAN_POINT ( 'NONE',  ( -33.99999999999998579, 6.180736333215580025, 0.000000000000000000 ) ) ;
#7372=DIRECTION ( 'NONE',  ( -1.000000000000000000, 1.084202172485504927E-16, 0.000000000000000000 ) ) ;
#7380=DIRECTION ( 'NONE',  ( -1.000000000000000000, 1.301042606982605814E-16, 0.000000000000000000 ) ) ;
#7394=LINE ( 'NONE', #5672, #11385 ) ;
#7443=FACE_OUTER_BOUND ( 'NONE', #7565, .T. ) ;
#7466=AXIS2_PLACEMENT_3D ( 'NONE', #7533, #7871, #7755 ) ;
#7492=CIRCLE ( 'NONE', #12197, 3.999999999999996447 ) ;
#7509=FACE_OUTER_BOUND ( 'NONE', #7584, .T. ) ;
#7518=DIRECTION ( 'NONE',  ( -1.000000000000000000, 1.264902534566437206E-16, 0.000000000000000000 ) ) ;
#7533=CARTESIAN_POINT ( 'NONE',  ( -13.85640646055084702, 1.500000000000008216, 7.999999999999705125 ) ) ;
#7538=DIRECTION ( 'NONE',  ( -1.000000000000000000, 1.020425574104004369E-16, 0.000000000000000000 ) ) ;
#7551=CARTESIAN_POINT ( 'NONE',  ( 7.310544252644470693E-15, 28.19616000222403684, 0.000000000000000000 ) ) ;
#7558=DIRECTION ( 'NONE',  ( -1.000000000000000000, 1.084202172485504434E-16, 0.000000000000000000 ) ) ;
#7559=AXIS2_PLACEMENT_3D ( 'NONE', #19420, #12747, #610 ) ;
#7565=EDGE_LOOP ( 'NONE', ( #14703, #8828, #2530, #21570 ) ) ;
#7568=CARTESIAN_POINT ( 'NONE',  ( 7.310544252644470693E-15, 28.19616000222403684, 0.000000000000000000 ) ) ;
#7584=EDGE_LOOP ( 'NONE', ( #6312, #10404, #9483, #7831, #4540, #9189, #13316, #11715, #13750, #12289 ) ) ;
#7636=EDGE_CURVE ( 'NONE', #6902, #20227, #7394, .T. ) ;
#7694=LINE ( 'NONE', #21673, #3780 ) ;
#7715=ORIENTED_EDGE ( 'NONE', *, *, #10073, .T. ) ;
#7725=CIRCLE ( 'NONE', #20525, 19.99999999999999289 ) ;
#7732=EDGE_LOOP ( 'NONE', ( #21914, #13397, #15186, #1406 ) ) ;
#7734=DIRECTION ( 'NONE',  ( 1.296372316667914327E-16, 1.000000000000000000, -0.000000000000000000 ) ) ;
#7751=ORIENTED_EDGE ( 'NONE', *, *, #9752, .T. ) ;
#7755=DIRECTION ( 'NONE',  ( 1.000000000000000000, -1.084202172485504927E-16, 0.000000000000000000 ) ) ;
#7756=DIRECTION ( 'NONE',  ( 1.296372316667914327E-16, 1.000000000000000000, -0.000000000000000000 ) ) ;
#7822=VECTOR ( 'NONE', #157, 1000.000000000000000 ) ;
#7831=ORIENTED_EDGE ( 'NONE', *, *, #13981, .T. ) ;
#7864=ORIENTED_EDGE ( 'NONE', *, *, #22665, .F. ) ;
#7865=EDGE_CURVE ( 'NONE', #18519, #15720, #480, .T. ) ;
#7871=DIRECTION ( 'NONE',  ( -1.296372316667914327E-16, -1.000000000000000000, 0.000000000000000000 ) ) ;
#7881=CARTESIAN_POINT ( 'NONE',  ( -10.39230484541309174, -25.00000000000000000, 5.999999999999708677 ) ) ;
#7883=CARTESIAN_POINT ( 'NONE',  ( -33.99999999999998579, 28.19616000222404040, 0.000000000000000000 ) ) ;
#7896=VECTOR ( 'NONE', #11080, 1000.000000000000000 ) ;
#7904=VERTEX_POINT ( 'NONE', #7364 ) ;
#7914=AXIS2_PLACEMENT_3D ( 'NONE', #16486, #793, #21765 ) ;
#7921=ORIENTED_EDGE ( 'NONE', *, *, #2630, .F. ) ;
#7943=VECTOR ( 'NONE', #354, 1000.000000000000000 ) ;
#7946=VERTEX_POINT ( 'NONE', #14678 ) ;
#7971=DIRECTION ( 'NONE',  ( 1.296372316667914327E-16, 1.000000000000000000, -0.000000000000000000 ) ) ;
#7986=CIRCLE ( 'NONE', #8353, 19.99999999999999289 ) ;
#8035=ORIENTED_EDGE ( 'NONE', *, *, #20864, .F. ) ;
#8039=PRODUCT ( 'FLYWHEEL', 'FLYWHEEL', '', ( #19144 ) ) ;
#8042=MECHANICAL_DESIGN_GEOMETRIC_PRESENTATION_REPRESENTATION('',(#2575),#11342);
#8065=VERTEX_POINT ( 'NONE', #9644 ) ;
#8079=VERTEX_POINT ( 'NONE', #4614 ) ;
#8140=DIRECTION ( 'NONE',  ( 0.000000000000000000, 0.000000000000000000, 1.000000000000000000 ) ) ;
#8188=DIRECTION ( 'NONE',  ( -1.000000000000000000, 1.371829164384562918E-16, 0.000000000000000000 ) ) ;
#8190=VERTEX_POINT ( 'NONE', #15352 ) ;
#8192=CARTESIAN_POINT ( 'NONE',  ( 13.85640646055130709, -1.500000000000015099, -8.000000000000097700 ) ) ;
#8209=EDGE_CURVE ( 'NONE', #17260, #651, #7310, .T. ) ;
#8214=CARTESIAN_POINT ( 'NONE',  ( -13.85640646055084702, -25.00000000000000000, 11.99999999999970335 ) ) ;
#8244=VECTOR ( 'NONE', #3771, 1000.000000000000114 ) ;
#8288=ADVANCED_FACE ( 'NONE', ( #7443 ), #21549, .F. ) ;
#8296=CARTESIAN_POINT ( 'NONE',  ( 12.00000000000000355, 1.500000000000003553, 0.000000000000000000 ) ) ;
#8312=ADVANCED_FACE ( 'NONE', ( #12260 ), #5390, .F. ) ;
#8320=ORIENTED_EDGE ( 'NONE', *, *, #18843, .F. ) ;
#8323=VECTOR ( 'NONE', #19272, 1000.000000000000000 ) ;
#8338=EDGE_LOOP ( 'NONE', ( #2449, #8407, #20845, #3103 ) ) ;
#8353=AXIS2_PLACEMENT_3D ( 'NONE', #17451, #15386, #5106 ) ;
#8372=AXIS2_PLACEMENT_3D ( 'NONE', #4392, #22030, #11368 ) ;
#8407=ORIENTED_EDGE ( 'NONE', *, *, #2380, .T. ) ;
#8408=DIRECTION ( 'NONE',  ( 1.296372316667914327E-16, 1.000000000000000000, -0.000000000000000000 ) ) ;
#8446=CARTESIAN_POINT ( 'NONE',  ( -10.00000000000000000, -4.824555320336763486, 3.000000000000000000 ) ) ;
#8458=ORIENTED_EDGE ( 'NONE', *, *, #5450, .T. ) ;
#8531=CARTESIAN_POINT ( 'NONE',  ( 4.238639668822796917E-15, 4.500000000000007105, 0.000000000000000000 ) ) ;
#8535=AXIS2_PLACEMENT_3D ( 'NONE', #9445, #15960, #10801 ) ;
#8540=ORIENTED_EDGE ( 'NONE', *, *, #5450, .F. ) ;
#8551=CARTESIAN_POINT ( 'NONE',  ( 19.99999999999999645, 1.500000000000009104, 2.449293598294705724E-15 ) ) ;
#8558=ORIENTED_EDGE ( 'NONE', *, *, #13729, .F. ) ;
#8581=CARTESIAN_POINT ( 'NONE',  ( 19.99999999999999645, -4.500000000000013323, 0.000000000000000000 ) ) ;
#8583=PLANE ( 'NONE',  #17085 ) ;
#8614=DIRECTION ( 'NONE',  ( -0.9659258262890680902, -0.2588190451025216832, 1.182917971378669349E-16 ) ) ;
#8629=ORIENTED_EDGE ( 'NONE', *, *, #7865, .T. ) ;
#8630=DIRECTION ( 'NONE',  ( -1.000000000000000000, 1.275531967630005492E-16, 0.000000000000000000 ) ) ;
#8634=VERTEX_POINT ( 'NONE', #21400 ) ;
#8667=ORIENTED_EDGE ( 'NONE', *, *, #4580, .F. ) ;
#8683=VERTEX_POINT ( 'NONE', #10614 ) ;
#8731=CIRCLE ( 'NONE', #14569, 11.99999999999985434 ) ;
#8735=CARTESIAN_POINT ( 'NONE',  ( -34.00000000000000000, -6.180736333215561373, 4.163799117101000559E-15 ) ) ;
#8780=EDGE_LOOP ( 'NONE', ( #18041, #12027, #15488, #6244 ) ) ;
#8790=DIRECTION ( 'NONE',  ( -0.9659258262890679791, 0.2588190451025219052, 0.000000000000000000 ) ) ;
#8809=CYLINDRICAL_SURFACE ( 'NONE', #19635, 33.99999999999999289 ) ;
#8819=DIRECTION ( 'NONE',  ( -1.000000000000000000, 1.264902534566421429E-16, 0.000000000000000000 ) ) ;
#8828=ORIENTED_EDGE ( 'NONE', *, *, #10657, .F. ) ;
#8832=DIRECTION ( 'NONE',  ( 1.296372316667914327E-16, 1.000000000000000000, -0.000000000000000000 ) ) ;
#8852=ORIENTED_EDGE ( 'NONE', *, *, #8209, .T. ) ;
#8889=LINE ( 'NONE', #10707, #970 ) ;
#8891=DIRECTION ( 'NONE',  ( -1.296372316667914327E-16, -1.000000000000000000, 0.000000000000000000 ) ) ;
#8937=DIRECTION ( 'NONE',  ( 1.296372316667914327E-16, 1.000000000000000000, -0.000000000000000000 ) ) ;
#8950=ORIENTED_EDGE ( 'NONE', *, *, #4299, .T. ) ;
#8956=AXIS2_PLACEMENT_3D ( 'NONE', #18291, #9579, #18640 ) ;
#8968=ORIENTED_EDGE ( 'NONE', *, *, #5114, .T. ) ;
#8971=EDGE_CURVE ( 'NONE', #7032, #4351, #3827, .T. ) ;
#8978=DIRECTION ( 'NONE',  ( 1.296372316667914327E-16, 1.000000000000000000, -0.000000000000000000 ) ) ;
#8991=EDGE_CURVE ( 'NONE', #9647, #2304, #17079, .T. ) ;
#9005=DIRECTION ( 'NONE',  ( 1.296372316667914327E-16, 1.000000000000000000, -0.000000000000000000 ) ) ;
#9034=CARTESIAN_POINT ( 'NONE',  ( -19.99999999999998579, 28.19616000222404040, 0.000000000000000000 ) ) ;
#9095=CIRCLE ( 'NONE', #21910, 11.99999999999985434 ) ;
#9110=CONICAL_SURFACE ( 'NONE', #8372, 19.99999999999999289, 1.308996938995746984 ) ;
#9114=VERTEX_POINT ( 'NONE', #22147 ) ;
#9125=LINE ( 'NONE', #1808, #14169 ) ;
#9134=EDGE_CURVE ( 'NONE', #5841, #11067, #17464, .T. ) ;
#9139=FACE_OUTER_BOUND ( 'NONE', #22418, .T. ) ;
#9152=DIRECTION ( 'NONE',  ( 0.000000000000000000, 0.000000000000000000, -1.000000000000000000 ) ) ;
#9155=ORIENTED_EDGE ( 'NONE', *, *, #22665, .T. ) ;
#9172=LINE ( 'NONE', #14547, #10803 ) ;
#9187=ORIENTED_EDGE ( 'NONE', *, *, #18035, .T. ) ;
#9189=ORIENTED_EDGE ( 'NONE', *, *, #13218, .T. ) ;
#9193=DIRECTION ( 'NONE',  ( -1.296372316667914327E-16, -1.000000000000000000, 0.000000000000000000 ) ) ;
#9219=ORIENTED_EDGE ( 'NONE', *, *, #19365, .T. ) ;
#9226=CARTESIAN_POINT ( 'NONE',  ( 4.238639668822796917E-15, 4.500000000000007105, 0.000000000000000000 ) ) ;
#9227=VERTEX_POINT ( 'NONE', #7008 ) ;
#9234=CARTESIAN_POINT ( 'NONE',  ( -8.485281374238564212, 1.499999999999997558, 3.000000000000000000 ) ) ;
#9241=DIRECTION ( 'NONE',  ( 1.000000000000000000, -1.296372316667914327E-16, 0.000000000000000000 ) ) ;
#9263=AXIS2_PLACEMENT_3D ( 'NONE', #5904, #12872, #286 ) ;
#9277=DIRECTION ( 'NONE',  ( 1.296372316667914327E-16, 1.000000000000000000, -0.000000000000000000 ) ) ;
#9300=DIRECTION ( 'NONE',  ( -1.000000000000000000, 1.084202172485504434E-16, 0.000000000000000000 ) ) ;
#9303=VERTEX_POINT ( 'NONE', #11002 ) ;
#9306=( NAMED_UNIT ( * ) PLANE_ANGLE_UNIT ( ) SI_UNIT ( $, .RADIAN. ) );
#9311=CARTESIAN_POINT ( 'NONE',  ( 2.854018578421813982E-15, -6.180736333215565814, 0.000000000000000000 ) ) ;
#9319=DIRECTION ( 'NONE',  ( 1.296372316667914327E-16, 1.000000000000000000, -0.000000000000000000 ) ) ;
#9344=DIRECTION ( 'NONE',  ( -1.296372316667914327E-16, -1.000000000000000000, 0.000000000000000000 ) ) ;
#9367=AXIS2_PLACEMENT_3D ( 'NONE', #3778, #10741, #10861 ) ;
#9445=CARTESIAN_POINT ( 'NONE',  ( 4.724946350300523916E-15, 8.251288694035745053, 0.000000000000000000 ) ) ;
#9451=EDGE_CURVE ( 'NONE', #12869, #626, #20061, .T. ) ;
#9464=AXIS2_PLACEMENT_3D ( 'NONE', #10950, #9005, #298 ) ;
#9466=FACE_OUTER_BOUND ( 'NONE', #1661, .T. ) ;
#9482=ORIENTED_EDGE ( 'NONE', *, *, #6271, .F. ) ;
#9483=ORIENTED_EDGE ( 'NONE', *, *, #6684, .F. ) ;
#9484=EDGE_CURVE ( 'NONE', #8190, #1985, #5960, .T. ) ;
#9499=CARTESIAN_POINT ( 'NONE',  ( 4.044183821322609990E-15, 3.000000000000006217, 0.000000000000000000 ) ) ;
#9541=DIRECTION ( 'NONE',  ( 1.000000000000000000, -1.084202172485504927E-16, 0.000000000000000000 ) ) ;
#9542=DIRECTION ( 'NONE',  ( -0.000000000000000000, 1.000000000000000000, -0.000000000000000000 ) ) ;
#9573=ORIENTED_EDGE ( 'NONE', *, *, #3565, .T. ) ;
#9579=DIRECTION ( 'NONE',  ( 1.296372316667914327E-16, 1.000000000000000000, -0.000000000000000000 ) ) ;
#9586=DIRECTION ( 'NONE',  ( -0.000000000000000000, 1.000000000000000000, -0.000000000000000000 ) ) ;
#9644=CARTESIAN_POINT ( 'NONE',  ( 6.383438919230843859E-14, 1.500000000000015099, -20.00000000000029488 ) ) ;
#9647=VERTEX_POINT ( 'NONE', #780 ) ;
#9702=AXIS2_PLACEMENT_3D ( 'NONE', #12268, #3467, #14195 ) ;
#9712=ORIENTED_EDGE ( 'NONE', *, *, #549, .T. ) ;
#9732=CIRCLE ( 'NONE', #1326, 19.99999999999999289 ) ;
#9747=CARTESIAN_POINT ( 'NONE',  ( 3.877306978638209416E-14, -25.00000000000000000, -12.00000000000000355 ) ) ;
#9752=EDGE_CURVE ( 'NONE', #5947, #19486, #3303, .T. ) ;
#9778=LINE ( 'NONE', #13297, #22085 ) ;
#9779=CIRCLE ( 'NONE', #6798, 33.99999999999999289 ) ;
#9797=CARTESIAN_POINT ( 'NONE',  ( 34.00000000000000000, -6.180736333215569367, 0.000000000000000000 ) ) ;
#9816=AXIS2_PLACEMENT_3D ( 'NONE', #19556, #5238, #3859 ) ;
#9821=CARTESIAN_POINT ( 'NONE',  ( -10.00000000000000000, 1.499999999999997780, -3.000000000000000000 ) ) ;
#9832=VECTOR ( 'NONE', #12749, 1000.000000000000227 ) ;
#9854=ADVANCED_FACE ( 'NONE', ( #20589 ), #17145, .F. ) ;
#9900=ORIENTED_EDGE ( 'NONE', *, *, #2402, .T. ) ;
#9913=LINE ( 'NONE', #16904, #14463 ) ;
#9918=ADVANCED_FACE ( 'NONE', ( #5681 ), #2137, .F. ) ;
#9991=EDGE_CURVE ( 'NONE', #2304, #13173, #15659, .T. ) ;
#9993=CARTESIAN_POINT ( 'NONE',  ( 7.310544252644470693E-15, 28.19616000222403684, 0.000000000000000000 ) ) ;
#9997=AXIS2_PLACEMENT_3D ( 'NONE', #16395, #2307, #9300 ) ;
#10001=DIRECTION ( 'NONE',  ( 1.000000000000000000, -1.296372316667914327E-16, 0.000000000000000000 ) ) ;
#10006=EDGE_CURVE ( 'NONE', #626, #5224, #1384, .T. ) ;
#10020=EDGE_CURVE ( 'NONE', #3259, #7904, #9125, .T. ) ;
#10037=DIRECTION ( 'NONE',  ( 1.296372316667914327E-16, 1.000000000000000000, -0.000000000000000000 ) ) ;
#10052=ORIENTED_EDGE ( 'NONE', *, *, #20864, .T. ) ;
#10057=CONICAL_SURFACE ( 'NONE', #1663, 22.12933039895921539, 1.308996938995746095 ) ;
#10064=LINE ( 'NONE', #3334, #518 ) ;
#10073=EDGE_CURVE ( 'NONE', #18457, #8634, #669, .T. ) ;
#10081=CARTESIAN_POINT ( 'NONE',  ( 10.39230484541308819, -25.00000000000000000, 6.000000000000008882 ) ) ;
#10111=ORIENTED_EDGE ( 'NONE', *, *, #19975, .F. ) ;
#10136=ORIENTED_EDGE ( 'NONE', *, *, #501, .F. ) ;
#10142=CYLINDRICAL_SURFACE ( 'NONE', #656, 33.99999999999999289 ) ;
#10159=CYLINDRICAL_SURFACE ( 'NONE', #2369, 4.000000000000000000 ) ;
#10216=EDGE_LOOP ( 'NONE', ( #8540, #19843, #16933, #7143 ) ) ;
#10253=EDGE_CURVE ( 'NONE', #22196, #4403, #13786, .T. ) ;
#10275=PLANE ( 'NONE',  #3161 ) ;
#10321=DIRECTION ( 'NONE',  ( -0.000000000000000000, 1.000000000000000000, -0.000000000000000000 ) ) ;
#10323=DIRECTION ( 'NONE',  ( 1.296372316667914327E-16, 1.000000000000000000, -0.000000000000000000 ) ) ;
#10327=AXIS2_PLACEMENT_3D ( 'NONE', #22634, #1650, #8630 ) ;
#10351=CIRCLE ( 'NONE', #21336, 4.000000000000000000 ) ;
#10352=AXIS2_PLACEMENT_3D ( 'NONE', #3367, #10323, #1638 ) ;
#10354=LINE ( 'NONE', #19084, #7822 ) ;
#10382=CIRCLE ( 'NONE', #21381, 4.000000000000000000 ) ;
#10404=ORIENTED_EDGE ( 'NONE', *, *, #22691, .T. ) ;
#10415=DIRECTION ( 'NONE',  ( -1.000000000000000000, 1.445602896647339410E-16, 0.000000000000000000 ) ) ;
#10421=CARTESIAN_POINT ( 'NONE',  ( -10.00000000000000000, 1.499999999999997780, -3.000000000000000000 ) ) ;
#10428=LINE ( 'NONE', #17426, #1682 ) ;
#10432=EDGE_CURVE ( 'NONE', #21559, #11580, #10382, .T. ) ;
#10446=ORIENTED_EDGE ( 'NONE', *, *, #22691, .F. ) ;
#10459=AXIS2_PLACEMENT_3D ( 'NONE', #20741, #7201, #19024 ) ;
#10484=ORIENTED_EDGE ( 'NONE', *, *, #10697, .T. ) ;
#10491=ADVANCED_FACE ( 'NONE', ( #16617 ), #925, .F. ) ;
#10555=ORIENTED_EDGE ( 'NONE', *, *, #10253, .F. ) ;
#10579=EDGE_CURVE ( 'NONE', #11067, #17027, #10064, .T. ) ;
#10585=CARTESIAN_POINT ( 'NONE',  ( 3.460816278822046447E-15, -1.500000000000011768, 0.000000000000000000 ) ) ;
#10607=DIRECTION ( 'NONE',  ( 1.296372316667914327E-16, 1.000000000000000000, -0.000000000000000000 ) ) ;
#10614=CARTESIAN_POINT ( 'NONE',  ( 4.000000000000003553, 1.499999999999994005, 4.898587196589412829E-16 ) ) ;
#10634=EDGE_LOOP ( 'NONE', ( #15005, #1375, #946, #7211 ) ) ;
#10657=EDGE_CURVE ( 'NONE', #16002, #12869, #7492, .T. ) ;
#10668=ORIENTED_EDGE ( 'NONE', *, *, #1892, .F. ) ;
#10671=FACE_OUTER_BOUND ( 'NONE', #4696, .T. ) ;
#10675=VERTEX_POINT ( 'NONE', #14400 ) ;
#10692=ORIENTED_EDGE ( 'NONE', *, *, #4580, .T. ) ;
#10697=EDGE_CURVE ( 'NONE', #18519, #22383, #17738, .T. ) ;
#10702=CIRCLE ( 'NONE', #11804, 11.99999999999999822 ) ;
#10707=CARTESIAN_POINT ( 'NONE',  ( -9.999999999999998224, 12.49999999999999822, 3.000000000000000000 ) ) ;
#10716=VERTEX_POINT ( 'NONE', #17966 ) ;
#10741=DIRECTION ( 'NONE',  ( -1.296372316667914327E-16, -1.000000000000000000, 0.000000000000000000 ) ) ;
#10747=ADVANCED_FACE ( 'NONE', ( #21250 ), #5595, .F. ) ;
#10751=CARTESIAN_POINT ( 'NONE',  ( 7.310544252644470693E-15, 28.19616000222403684, 0.000000000000000000 ) ) ;
#10768=EDGE_CURVE ( 'NONE', #5161, #8683, #10351, .T. ) ;
#10801=DIRECTION ( 'NONE',  ( -1.000000000000000000, 1.530638361156006492E-16, 0.000000000000000000 ) ) ;
#10803=VECTOR ( 'NONE', #21664, 1000.000000000000000 ) ;
#10861=DIRECTION ( 'NONE',  ( 1.000000000000000000, -1.296372316667914327E-16, 0.000000000000000000 ) ) ;
#10889=DIRECTION ( 'NONE',  ( 1.000000000000000000, -1.084202172485504434E-16, 0.000000000000000000 ) ) ;
#10893=EDGE_CURVE ( 'NONE', #21392, #9227, #9778, .T. ) ;
#10940=EDGE_CURVE ( 'NONE', #18457, #15515, #20890, .T. ) ;
#10943=ORIENTED_EDGE ( 'NONE', *, *, #20503, .F. ) ;
#10949=PRODUCT_DEFINITION_CONTEXT ( 'detailed design', #11506, 'design' ) ;
#10950=CARTESIAN_POINT ( 'NONE',  ( 7.310544252644470693E-15, 28.19616000222403684, 0.000000000000000000 ) ) ;
#10980=CARTESIAN_POINT ( 'NONE',  ( 10.39230484541330846, -1.500000000000015099, -5.999999999999929834 ) ) ;
#10985=CYLINDRICAL_SURFACE ( 'NONE', #11142, 34.00000000000000000 ) ;
#11002=CARTESIAN_POINT ( 'NONE',  ( -17.32050807568873196, 1.500000000000015099, 9.999999999999772626 ) ) ;
#11061=CIRCLE ( 'NONE', #22427, 34.00000000000000000 ) ;
#11064=EDGE_CURVE ( 'NONE', #9114, #11241, #13387, .T. ) ;
#11067=VERTEX_POINT ( 'NONE', #2424 ) ;
#11080=DIRECTION ( 'NONE',  ( 1.296372316667914327E-16, 1.000000000000000000, -0.000000000000000000 ) ) ;
#11104=CARTESIAN_POINT ( 'NONE',  ( 4.724946350300523916E-15, 8.251288694035745053, 0.000000000000000000 ) ) ;
#11116=ORIENTED_EDGE ( 'NONE', *, *, #10432, .F. ) ;
#11136=DIRECTION ( 'NONE',  ( 1.296372316667914327E-16, 1.000000000000000000, -0.000000000000000000 ) ) ;
#11137=ORIENTED_EDGE ( 'NONE', *, *, #19365, .F. ) ;
#11142=AXIS2_PLACEMENT_3D ( 'NONE', #7551, #4354, #5941 ) ;
#11202=FACE_OUTER_BOUND ( 'NONE', #17330, .T. ) ;
#11213=CYLINDRICAL_SURFACE ( 'NONE', #20028, 3.999999999999998224 ) ;
#11232=DIRECTION ( 'NONE',  ( -1.000000000000000000, 1.301042606982605814E-16, 0.000000000000000000 ) ) ;
#11240=VECTOR ( 'NONE', #4475, 1000.000000000000000 ) ;
#11241=VERTEX_POINT ( 'NONE', #17064 ) ;
#11253=CARTESIAN_POINT ( 'NONE',  ( -10.00000000000000000, -4.824555320336763486, -3.000000000000000000 ) ) ;
#11276=ORIENTED_EDGE ( 'NONE', *, *, #9484, .T. ) ;
#11287=DIRECTION ( 'NONE',  ( 0.000000000000000000, 0.000000000000000000, 1.000000000000000000 ) ) ;
#11342=( GEOMETRIC_REPRESENTATION_CONTEXT ( 3 ) GLOBAL_UNCERTAINTY_ASSIGNED_CONTEXT ( ( #4407 ) ) GLOBAL_UNIT_ASSIGNED_CONTEXT ( ( #180, #20943, #15764 ) ) REPRESENTATION_CONTEXT ( 'NONE', 'WORKASPACE' ) );
#11368=DIRECTION ( 'NONE',  ( 1.000000000000000000, -1.301042606982605814E-16, 0.000000000000000000 ) ) ;
#11385=VECTOR ( 'NONE', #12647, 1000.000000000000000 ) ;
#11394=AXIS2_PLACEMENT_3D ( 'NONE', #6773, #13737, #10415 ) ;
#11412=ORIENTED_EDGE ( 'NONE', *, *, #8991, .T. ) ;
#11435=ADVANCED_FACE ( 'NONE', ( #20154 ), #16361, .F. ) ;
#11450=CARTESIAN_POINT ( 'NONE',  ( -9.999999999999998224, 12.49999999999999822, -3.000000000000000000 ) ) ;
#11479=DIRECTION ( 'NONE',  ( 1.296372316667914327E-16, 1.000000000000000000, -0.000000000000000000 ) ) ;
#11505=ORIENTED_EDGE ( 'NONE', *, *, #2745, .T. ) ;
#11506=APPLICATION_CONTEXT ( 'automotive_design' ) ;
#11511=ORIENTED_EDGE ( 'NONE', *, *, #15443, .T. ) ;
#11533=EDGE_LOOP ( 'NONE', ( #5214, #14667, #7244, #17815 ) ) ;
#11544=DIRECTION ( 'NONE',  ( -0.000000000000000000, 1.000000000000000000, -0.000000000000000000 ) ) ;
#11555=FACE_OUTER_BOUND ( 'NONE', #212, .T. ) ;
#11580=VERTEX_POINT ( 'NONE', #11974 ) ;
#11581=DIRECTION ( 'NONE',  ( 1.000000000000000000, -1.275531967630005245E-16, 0.000000000000000000 ) ) ;
#11584=AXIS2_PLACEMENT_3D ( 'NONE', #14912, #18022, #2683 ) ;
#11617=ORIENTED_EDGE ( 'NONE', *, *, #19164, .F. ) ;
#11628=DIRECTION ( 'NONE',  ( -1.000000000000000000, 1.084202172485505420E-16, 0.000000000000000000 ) ) ;
#11639=VECTOR ( 'NONE', #17112, 1000.000000000000000 ) ;
#11643=AXIS2_PLACEMENT_3D ( 'NONE', #18284, #2821, #2362 ) ;
#11664=AXIS2_PLACEMENT_3D ( 'NONE', #17219, #13883, #5201 ) ;
#11670=VERTEX_POINT ( 'NONE', #1788 ) ;
#11673=EDGE_LOOP ( 'NONE', ( #8320, #2044, #5923, #11511, #627, #21073, #676, #17999 ) ) ;
#11676=ORIENTED_EDGE ( 'NONE', *, *, #3163, .T. ) ;
#11706=ORIENTED_EDGE ( 'NONE', *, *, #10020, .F. ) ;
#11715=ORIENTED_EDGE ( 'NONE', *, *, #19975, .T. ) ;
#11722=AXIS2_PLACEMENT_3D ( 'NONE', #5984, #9193, #18010 ) ;
#11749=ORIENTED_EDGE ( 'NONE', *, *, #13729, .T. ) ;
#11801=ORIENTED_EDGE ( 'NONE', *, *, #16452, .F. ) ;
#11804=AXIS2_PLACEMENT_3D ( 'NONE', #15092, #19937, #6191 ) ;
#11831=CIRCLE ( 'NONE', #9997, 4.000000000000000000 ) ;
#11854=DIRECTION ( 'NONE',  ( -0.000000000000000000, 1.000000000000000000, -0.000000000000000000 ) ) ;
#11884=AXIS2_PLACEMENT_3D ( 'NONE', #3891, #9152, #2514 ) ;
#11913=EDGE_LOOP ( 'NONE', ( #1775, #11276, #4676, #20981 ) ) ;
#11923=DIRECTION ( 'NONE',  ( 1.296372316667914327E-16, 1.000000000000000000, -0.000000000000000000 ) ) ;
#11924=DIRECTION ( 'NONE',  ( -1.000000000000000000, 1.734723475976807834E-16, 0.000000000000000000 ) ) ;
#11932=CARTESIAN_POINT ( 'NONE',  ( 34.00000000000000000, -6.180736333215569367, 0.000000000000000000 ) ) ;
#11937=ORIENTED_EDGE ( 'NONE', *, *, #4182, .F. ) ;
#11974=CARTESIAN_POINT ( 'NONE',  ( -10.39230484541304911, 1.500000000000005773, -6.000000000000371259 ) ) ;
#11982=ADVANCED_FACE ( 'NONE', ( #6460 ), #3024, .T. ) ;
#12025=VECTOR ( 'NONE', #8408, 1000.000000000000000 ) ;
#12026=CARTESIAN_POINT ( 'NONE',  ( 13.85640646055118808, -25.00000000000000000, 7.999999999999710454 ) ) ;
#12027=ORIENTED_EDGE ( 'NONE', *, *, #21989, .T. ) ;
#12111=ADVANCED_FACE ( 'NONE', ( #1756, #19288 ), #19058, .F. ) ;
#12133=DIRECTION ( 'NONE',  ( 0.000000000000000000, 0.000000000000000000, 1.000000000000000000 ) ) ;
#12145=ORIENTED_EDGE ( 'NONE', *, *, #19378, .T. ) ;
#12155=LINE ( 'NONE', #6780, #8323 ) ;
#12164=CARTESIAN_POINT ( 'NONE',  ( -10.39230484541300825, -25.00000000000000000, -6.000000000000442313 ) ) ;
#12166=DIRECTION ( 'NONE',  ( -0.000000000000000000, 0.000000000000000000, 1.000000000000000000 ) ) ;
#12197=AXIS2_PLACEMENT_3D ( 'NONE', #21408, #5377, #19470 ) ;
#12199=DIRECTION ( 'NONE',  ( 1.296372316667914327E-16, 1.000000000000000000, -0.000000000000000000 ) ) ;
#12211=CARTESIAN_POINT ( 'NONE',  ( 3.266360431321861887E-15, -2.999999999999995559, 0.000000000000000000 ) ) ;
#12217=DIRECTION ( 'NONE',  ( 1.000000000000000000, -1.084202172485505420E-16, 0.000000000000000000 ) ) ;
#12241=EDGE_CURVE ( 'NONE', #16483, #10675, #11831, .T. ) ;
#12246=ORIENTED_EDGE ( 'NONE', *, *, #15530, .F. ) ;
#12251=EDGE_CURVE ( 'NONE', #15720, #15515, #7694, .T. ) ;
#12260=FACE_OUTER_BOUND ( 'NONE', #4665, .T. ) ;
#12268=CARTESIAN_POINT ( 'NONE',  ( 0.000000000000000000, -1.500000000000015099, 0.000000000000000000 ) ) ;
#12279=DIRECTION ( 'NONE',  ( -1.000000000000000000, 1.020425574104004122E-16, 0.000000000000000000 ) ) ;
#12289=ORIENTED_EDGE ( 'NONE', *, *, #4592, .F. ) ;
#12354=DIRECTION ( 'NONE',  ( 1.000000000000000000, -1.296372316667914327E-16, 0.000000000000000000 ) ) ;
#12363=AXIS2_PLACEMENT_3D ( 'NONE', #22014, #4147, #11232 ) ;
#12419=DIRECTION ( 'NONE',  ( -1.000000000000000000, 1.301042606982605814E-16, 0.000000000000000000 ) ) ;
#12440=CARTESIAN_POINT ( 'NONE',  ( 3.460816278822046447E-15, -1.500000000000011768, 0.000000000000000000 ) ) ;
#12449=DIRECTION ( 'NONE',  ( 0.9659258262890679791, 0.2588190451025219052, 1.182917971378669349E-16 ) ) ;
#12467=CIRCLE ( 'NONE', #6632, 4.000000000000000000 ) ;
#12497=CARTESIAN_POINT ( 'NONE',  ( 34.00000000000000000, 8.251288694035739724, 4.163799117100999770E-15 ) ) ;
#12514=CARTESIAN_POINT ( 'NONE',  ( 3.849727973822423851E-15, 1.500000000000011768, 0.000000000000000000 ) ) ;
#12530=ORIENTED_EDGE ( 'NONE', *, *, #22654, .F. ) ;
#12588=VERTEX_POINT ( 'NONE', #20863 ) ;
#12628=CARTESIAN_POINT ( 'NONE',  ( 3.849727973822423851E-15, 1.500000000000011768, 0.000000000000000000 ) ) ;
#12647=DIRECTION ( 'NONE',  ( 1.296372316667914327E-16, 1.000000000000000000, -0.000000000000000000 ) ) ;
#12649=ORIENTED_EDGE ( 'NONE', *, *, #18562, .F. ) ;
#12652=CIRCLE ( 'NONE', #7914, 34.00000000000000000 ) ;
#12664=CARTESIAN_POINT ( 'NONE',  ( -8.485281374238560659, 28.19616000222403684, 3.000000000000000000 ) ) ;
#12670=DIRECTION ( 'NONE',  ( -1.296372316667914327E-16, -1.000000000000000000, 0.000000000000000000 ) ) ;
#12698=AXIS2_PLACEMENT_3D ( 'NONE', #6438, #13401, #11924 ) ;
#12702=DIRECTION ( 'NONE',  ( 1.296372316667914327E-16, 1.000000000000000000, -0.000000000000000000 ) ) ;
#12712=FACE_OUTER_BOUND ( 'NONE', #13852, .T. ) ;
#12743=CARTESIAN_POINT ( 'NONE',  ( 0.000000000000000000, -1.500000000000015099, 11.99999999999985256 ) ) ;
#12747=DIRECTION ( 'NONE',  ( -1.296372316667914327E-16, -1.000000000000000000, 0.000000000000000000 ) ) ;
#12749=DIRECTION ( 'NONE',  ( 0.9659258262890680902, 0.2588190451025216832, 1.182917971378669349E-16 ) ) ;
#12753=DIRECTION ( 'NONE',  ( 1.296372316667914327E-16, 1.000000000000000000, -0.000000000000000000 ) ) ;
#12766=CARTESIAN_POINT ( 'NONE',  ( 3.460816278822046447E-15, -1.500000000000011768, 0.000000000000000000 ) ) ;
#12772=CIRCLE ( 'NONE', #2924, 19.99999999999999289 ) ;
#12798=DIRECTION ( 'NONE',  ( 1.296372316667914327E-16, 1.000000000000000000, -0.000000000000000000 ) ) ;
#12816=EDGE_CURVE ( 'NONE', #15720, #14743, #12652, .T. ) ;
#12832=VECTOR ( 'NONE', #5175, 1000.000000000000000 ) ;
#12833=ORIENTED_EDGE ( 'NONE', *, *, #10768, .T. ) ;
#12847=CARTESIAN_POINT ( 'NONE',  ( -3.999999999999996447, 1.499999999999994893, 0.000000000000000000 ) ) ;
#12866=ADVANCED_FACE ( 'NONE', ( #11555 ), #21078, .F. ) ;
#12869=VERTEX_POINT ( 'NONE', #902 ) ;
#12872=DIRECTION ( 'NONE',  ( -1.296372316667914327E-16, -1.000000000000000000, 0.000000000000000000 ) ) ;
#12961=DIRECTION ( 'NONE',  ( 1.296372316667914327E-16, 1.000000000000000000, -0.000000000000000000 ) ) ;
#12983=ADVANCED_FACE ( 'NONE', ( #19007, #4799 ), #10275, .F. ) ;
#12999=DIRECTION ( 'NONE',  ( 1.296372316667914327E-16, 1.000000000000000000, -0.000000000000000000 ) ) ;
#13055=VECTOR ( 'NONE', #2871, 1000.000000000000000 ) ;
#13061=ORIENTED_EDGE ( 'NONE', *, *, #2296, .T. ) ;
#13077=CIRCLE ( 'NONE', #2847, 19.99999999999999289 ) ;
#13129=CARTESIAN_POINT ( 'NONE',  ( 3.849727973822421485E-15, 1.499999999999994449, 0.000000000000000000 ) ) ;
#13149=AXIS2_PLACEMENT_3D ( 'NONE', #10751, #12702, #342 ) ;
#13173=VERTEX_POINT ( 'NONE', #2024 ) ;
#13188=EDGE_CURVE ( 'NONE', #19486, #4044, #16108, .T. ) ;
#13204=AXIS2_PLACEMENT_3D ( 'NONE', #21199, #9277, #7558 ) ;
#13218=EDGE_CURVE ( 'NONE', #11241, #11580, #21475, .T. ) ;
#13222=DIRECTION ( 'NONE',  ( -1.296372316667914327E-16, -1.000000000000000000, 0.000000000000000000 ) ) ;
#13229=DIRECTION ( 'NONE',  ( -1.000000000000000000, 1.020425574104004369E-16, 0.000000000000000000 ) ) ;
#13244=EDGE_CURVE ( 'NONE', #9303, #8079, #16709, .T. ) ;
#13251=DIRECTION ( 'NONE',  ( 0.000000000000000000, 0.000000000000000000, 1.000000000000000000 ) ) ;
#13282=EDGE_LOOP ( 'NONE', ( #18502, #13061 ) ) ;
#13297=CARTESIAN_POINT ( 'NONE',  ( 17.32050807568869644, -25.00000000000000000, 10.00000000000013323 ) ) ;
#13302=UNCERTAINTY_MEASURE_WITH_UNIT (LENGTH_MEASURE( 1.000000000000000082E-05 ), #598, 'distance_accuracy_value', 'NONE');
#13316=ORIENTED_EDGE ( 'NONE', *, *, #1012, .F. ) ;
#13319=ORIENTED_EDGE ( 'NONE', *, *, #15606, .F. ) ;
#13355=DIRECTION ( 'NONE',  ( 1.000000000000000000, -1.084202172485505420E-16, 0.000000000000000000 ) ) ;
#13364=ADVANCED_FACE ( 'NONE', ( #10671 ), #4654, .F. ) ;
#13387=LINE ( 'NONE', #9747, #1215 ) ;
#13397=ORIENTED_EDGE ( 'NONE', *, *, #5114, .F. ) ;
#13401=DIRECTION ( 'NONE',  ( 1.296372316667914327E-16, 1.000000000000000000, -0.000000000000000000 ) ) ;
#13436=LINE ( 'NONE', #9797, #11639 ) ;
#13450=CIRCLE ( 'NONE', #16026, 22.12933039895921539 ) ;
#13470=EDGE_CURVE ( 'NONE', #7904, #8190, #9779, .T. ) ;
#13530=ORIENTED_EDGE ( 'NONE', *, *, #7207, .T. ) ;
#13531=PLANE ( 'NONE',  #220 ) ;
#13556=VECTOR ( 'NONE', #3612, 1000.000000000000000 ) ;
#13572=ORIENTED_EDGE ( 'NONE', *, *, #10940, .T. ) ;
#13580=EDGE_LOOP ( 'NONE', ( #6811, #20221, #11505, #8950 ) ) ;
#13584=DIRECTION ( 'NONE',  ( 1.000000000000000000, -1.296372316667914327E-16, 0.000000000000000000 ) ) ;
#13620=EDGE_LOOP ( 'NONE', ( #10555, #5900, #10484, #20557, #14640, #15431, #3291, #9712 ) ) ;
#13684=DIRECTION ( 'NONE',  ( -0.000000000000000000, 1.000000000000000000, -0.000000000000000000 ) ) ;
#13704=CIRCLE ( 'NONE', #16956, 19.99999999999999289 ) ;
#13729=EDGE_CURVE ( 'NONE', #16483, #5161, #10428, .T. ) ;
#13737=DIRECTION ( 'NONE',  ( 1.296372316667914327E-16, 1.000000000000000000, -0.000000000000000000 ) ) ;
#13750=ORIENTED_EDGE ( 'NONE', *, *, #7636, .T. ) ;
#13765=EDGE_CURVE ( 'NONE', #7904, #7, #3583, .T. ) ;
#13779=ORIENTED_EDGE ( 'NONE', *, *, #17613, .F. ) ;
#13786=LINE ( 'NONE', #1436, #2511 ) ;
#13793=EDGE_CURVE ( 'NONE', #19871, #18308, #16357, .T. ) ;
#13827=ADVANCED_FACE ( 'NONE', ( #782 ), #19277, .T. ) ;
#13852=EDGE_LOOP ( 'NONE', ( #21637, #1918, #18770, #1649, #15295, #6583, #9900, #16591, #18384, #10692 ) ) ;
#13883=DIRECTION ( 'NONE',  ( 1.296372316667914327E-16, 1.000000000000000000, -0.000000000000000000 ) ) ;
#13899=CARTESIAN_POINT ( 'NONE',  ( 1.734786545154649763E-13, -1.500000000000015099, -16.00000000000029488 ) ) ;
#13930=ORIENTED_EDGE ( 'NONE', *, *, #14943, .T. ) ;
#13941=DIRECTION ( 'NONE',  ( -0.000000000000000000, 1.000000000000000000, -0.000000000000000000 ) ) ;
#13981=EDGE_CURVE ( 'NONE', #16002, #9114, #18152, .T. ) ;
#14010=ADVANCED_FACE ( 'NONE', ( #16020 ), #3446, .F. ) ;
#14016=DIRECTION ( 'NONE',  ( 1.296372316667914327E-16, 1.000000000000000000, -0.000000000000000000 ) ) ;
#14083=CARTESIAN_POINT ( 'NONE',  ( -10.00000000000000000, -4.824555320336763486, 3.000000000000000000 ) ) ;
#14089=CIRCLE ( 'NONE', #4633, 3.999999999999999112 ) ;
#14112=DIRECTION ( 'NONE',  ( -1.000000000000000000, 1.275531967630005492E-16, 0.000000000000000000 ) ) ;
#14125=ADVANCED_FACE ( 'NONE', ( #439 ), #10985, .T. ) ;
#14133=CARTESIAN_POINT ( 'NONE',  ( 3.849727973822421485E-15, 1.499999999999997780, 0.000000000000000000 ) ) ;
#14169=VECTOR ( 'NONE', #8790, 1000.000000000000000 ) ;
#14188=EDGE_CURVE ( 'NONE', #651, #21559, #14641, .T. ) ;
#14195=DIRECTION ( 'NONE',  ( -1.000000000000000000, 1.264902534566437453E-16, 0.000000000000000000 ) ) ;
#14255=ORIENTED_EDGE ( 'NONE', *, *, #397, .T. ) ;
#14273=ADVANCED_FACE ( 'NONE', ( #4798 ), #10159, .F. ) ;
#14314=LINE ( 'NONE', #122, #7943 ) ;
#14400=CARTESIAN_POINT ( 'NONE',  ( 4.000000000000003553, -1.500000000000015543, 4.898587196589412829E-16 ) ) ;
#14406=LINE ( 'NONE', #4014, #6165 ) ;
#14445=DIRECTION ( 'NONE',  ( 1.296372316667914327E-16, 1.000000000000000000, -0.000000000000000000 ) ) ;
#14463=VECTOR ( 'NONE', #11854, 1000.000000000000000 ) ;
#14474=ORIENTED_EDGE ( 'NONE', *, *, #12816, .F. ) ;
#14492=DIRECTION ( 'NONE',  ( 1.296372316667914327E-16, 1.000000000000000000, -0.000000000000000000 ) ) ;
#14494=DIRECTION ( 'NONE',  ( 1.296372316667914327E-16, 1.000000000000000000, -0.000000000000000000 ) ) ;
#14495=EDGE_CURVE ( 'NONE', #12869, #3845, #4599, .T. ) ;
#14533=CIRCLE ( 'NONE', #5774, 34.00000000000000000 ) ;
#14547=CARTESIAN_POINT ( 'NONE',  ( 9.000000000000005329, 12.49999999999999467, -3.000000000000000000 ) ) ;
#14562=VERTEX_POINT ( 'NONE', #11932 ) ;
#14569=AXIS2_PLACEMENT_3D ( 'NONE', #5014, #522, #7518 ) ;
#14582=LINE ( 'NONE', #5650, #9832 ) ;
#14640=ORIENTED_EDGE ( 'NONE', *, *, #13793, .F. ) ;
#14641=LINE ( 'NONE', #19925, #5302 ) ;
#14658=CYLINDRICAL_SURFACE ( 'NONE', #4231, 12.00000000000000000 ) ;
#14667=ORIENTED_EDGE ( 'NONE', *, *, #20503, .T. ) ;
#14668=FACE_OUTER_BOUND ( 'NONE', #17980, .T. ) ;
#14678=CARTESIAN_POINT ( 'NONE',  ( 6.383438919230843859E-14, -1.500000000000011768, -20.00000000000029488 ) ) ;
#14702=ORIENTED_EDGE ( 'NONE', *, *, #1505, .F. ) ;
#14703=ORIENTED_EDGE ( 'NONE', *, *, #9451, .F. ) ;
#14743=VERTEX_POINT ( 'NONE', #235 ) ;
#14806=CIRCLE ( 'NONE', #16655, 3.999999999999996447 ) ;
#14840=PLANE ( 'NONE',  #21142 ) ;
#14854=EDGE_CURVE ( 'NONE', #13173, #12588, #2961, .T. ) ;
#14878=CARTESIAN_POINT ( 'NONE',  ( -13.85640646055073333, -25.00000000000000000, -8.000000000000493827 ) ) ;
#14912=CARTESIAN_POINT ( 'NONE',  ( 2.585597902343947566E-15, -8.251288694035734395, 0.000000000000000000 ) ) ;
#14936=AXIS2_PLACEMENT_3D ( 'NONE', #8296, #20665, #10001 ) ;
#14943=EDGE_CURVE ( 'NONE', #14743, #14562, #16581, .T. ) ;
#14956=DIRECTION ( 'NONE',  ( -1.000000000000000000, 1.296372316667914327E-16, 0.000000000000000000 ) ) ;
#14983=AXIS2_PLACEMENT_3D ( 'NONE', #21619, #14494, #5685 ) ;
#14995=ORIENTED_EDGE ( 'NONE', *, *, #7865, .F. ) ;
#15005=ORIENTED_EDGE ( 'NONE', *, *, #16452, .T. ) ;
#15091=EDGE_CURVE ( 'NONE', #21392, #5486, #21435, .T. ) ;
#15092=CARTESIAN_POINT ( 'NONE',  ( 5.275737522157127195E-15, 12.49999999999999645, 0.000000000000000000 ) ) ;
#15186=ORIENTED_EDGE ( 'NONE', *, *, #3317, .F. ) ;
#15240=CARTESIAN_POINT ( 'NONE',  ( -3.418729828831206752E-14, -1.500000000000015099, 15.99999999999970512 ) ) ;
#15295=ORIENTED_EDGE ( 'NONE', *, *, #2659, .T. ) ;
#15310=CIRCLE ( 'NONE', #5452, 33.99999999999999289 ) ;
#15316=ORIENTED_EDGE ( 'NONE', *, *, #5012, .T. ) ;
#15347=SHAPE_DEFINITION_REPRESENTATION ( #4380, #21420 ) ;
#15352=CARTESIAN_POINT ( 'NONE',  ( 34.00000000000000000, 6.180736333215571143, 4.163799117100999770E-15 ) ) ;
#15358=CARTESIAN_POINT ( 'NONE',  ( 10.39230484541308819, -1.500000000000015099, 6.000000000000008882 ) ) ;
#15379=ORIENTED_EDGE ( 'NONE', *, *, #15600, .T. ) ;
#15386=DIRECTION ( 'NONE',  ( 1.296372316667914327E-16, 1.000000000000000000, -0.000000000000000000 ) ) ;
#15396=DIRECTION ( 'NONE',  ( -0.000000000000000000, 1.000000000000000000, -0.000000000000000000 ) ) ;
#15431=ORIENTED_EDGE ( 'NONE', *, *, #18035, .F. ) ;
#15443=EDGE_CURVE ( 'NONE', #3845, #10716, #9913, .T. ) ;
#15460=CYLINDRICAL_SURFACE ( 'NONE', #12698, 19.99999999999999289 ) ;
#15474=LINE ( 'NONE', #12164, #4914 ) ;
#15488=ORIENTED_EDGE ( 'NONE', *, *, #6797, .F. ) ;
#15491=DIRECTION ( 'NONE',  ( 0.000000000000000000, 0.000000000000000000, 1.000000000000000000 ) ) ;
#15504=DIRECTION ( 'NONE',  ( 1.296372316667914327E-16, 1.000000000000000000, -0.000000000000000000 ) ) ;
#15515=VERTEX_POINT ( 'NONE', #1664 ) ;
#15530=EDGE_CURVE ( 'NONE', #22383, #18308, #570, .T. ) ;
#15546=ORIENTED_EDGE ( 'NONE', *, *, #15443, .F. ) ;
#15600=EDGE_CURVE ( 'NONE', #8065, #21559, #9732, .T. ) ;
#15606=EDGE_CURVE ( 'NONE', #18457, #3259, #21353, .T. ) ;
#15659=CIRCLE ( 'NONE', #9816, 3.999999999999998224 ) ;
#15668=ORIENTED_EDGE ( 'NONE', *, *, #15091, .F. ) ;
#15669=CIRCLE ( 'NONE', #16786, 12.00000000000000000 ) ;
#15712=CARTESIAN_POINT ( 'NONE',  ( -3.999999999999996447, -1.500000000000014877, 0.000000000000000000 ) ) ;
#15720=VERTEX_POINT ( 'NONE', #16850 ) ;
#15738=CARTESIAN_POINT ( 'NONE',  ( -22.12933039895920828, 28.19616000222404040, 0.000000000000000000 ) ) ;
#15764=( NAMED_UNIT ( * ) SI_UNIT ( $, .STERADIAN. ) SOLID_ANGLE_UNIT ( ) );
#15797=CARTESIAN_POINT ( 'NONE',  ( 13.85640646055130709, -25.00000000000000000, -8.000000000000097700 ) ) ;
#15805=EDGE_CURVE ( 'NONE', #19486, #4351, #6833, .T. ) ;
#15840=ADVANCED_FACE ( 'NONE', ( #5271 ), #15896, .F. ) ;
#15896=CYLINDRICAL_SURFACE ( 'NONE', #10459, 3.999999999999998224 ) ;
#15899=ORIENTED_EDGE ( 'NONE', *, *, #4622, .F. ) ;
#15923=DIRECTION ( 'NONE',  ( 1.000000000000000000, 0.000000000000000000, 0.000000000000000000 ) ) ;
#15938=SHAPE_REPRESENTATION_RELATIONSHIP ( 'NONE' , 'NONE' ,  #21420, #6071 ) ;
#15947=LINE ( 'NONE', #21127, #13556 ) ;
#15960=DIRECTION ( 'NONE',  ( 1.296372316667914327E-16, 1.000000000000000000, -0.000000000000000000 ) ) ;
#16002=VERTEX_POINT ( 'NONE', #10980 ) ;
#16012=ADVANCED_FACE ( 'NONE', ( #7321 ), #19581, .F. ) ;
#16020=FACE_OUTER_BOUND ( 'NONE', #19650, .T. ) ;
#16026=AXIS2_PLACEMENT_3D ( 'NONE', #20458, #7971, #8188 ) ;
#16028=ADVANCED_FACE ( 'NONE', ( #11202 ), #10057, .T. ) ;
#16035=ORIENTED_EDGE ( 'NONE', *, *, #14188, .T. ) ;
#16069=LINE ( 'NONE', #19861, #272 ) ;
#16108=LINE ( 'NONE', #12664, #18542 ) ;
#16109=ORIENTED_EDGE ( 'NONE', *, *, #9451, .T. ) ;
#16112=LINE ( 'NONE', #18182, #512 ) ;
#16117=EDGE_CURVE ( 'NONE', #10716, #626, #14806, .T. ) ;
#16138=ORIENTED_EDGE ( 'NONE', *, *, #12816, .T. ) ;
#16178=DIRECTION ( 'NONE',  ( 1.296372316667914327E-16, 1.000000000000000000, -0.000000000000000000 ) ) ;
#16262=ORIENTED_EDGE ( 'NONE', *, *, #16117, .F. ) ;
#16357=LINE ( 'NONE', #4004, #22545 ) ;
#16361=CYLINDRICAL_SURFACE ( 'NONE', #21739, 4.000000000000145661 ) ;
#16395=CARTESIAN_POINT ( 'NONE',  ( 3.460816278822046447E-15, -1.500000000000015099, 0.000000000000000000 ) ) ;
#16401=ORIENTED_EDGE ( 'NONE', *, *, #19378, .F. ) ;
#16441=CARTESIAN_POINT ( 'NONE',  ( 7.310544252644470693E-15, 28.19616000222403684, 0.000000000000000000 ) ) ;
#16452=EDGE_CURVE ( 'NONE', #4044, #7032, #931, .T. ) ;
#16465=DIRECTION ( 'NONE',  ( -0.000000000000000000, 1.000000000000000000, -0.000000000000000000 ) ) ;
#16476=DIRECTION ( 'NONE',  ( 1.296372316667914327E-16, 1.000000000000000000, -0.000000000000000000 ) ) ;
#16481=CARTESIAN_POINT ( 'NONE',  ( -3.418729828831206752E-14, -25.00000000000000000, 15.99999999999970512 ) ) ;
#16483=VERTEX_POINT ( 'NONE', #15712 ) ;
#16486=CARTESIAN_POINT ( 'NONE',  ( 2.585597902343947566E-15, -8.251288694035734395, 0.000000000000000000 ) ) ;
#16524=DIRECTION ( 'NONE',  ( -1.296372316667914327E-16, -1.000000000000000000, 0.000000000000000000 ) ) ;
#16564=AXIS2_PLACEMENT_3D ( 'NONE', #12766, #18162, #5789 ) ;
#16567=DIRECTION ( 'NONE',  ( -1.000000000000000000, 1.301042606982605814E-16, 0.000000000000000000 ) ) ;
#16574=CIRCLE ( 'NONE', #9263, 3.999999999999998224 ) ;
#16581=LINE ( 'NONE', #888, #5348 ) ;
#16591=ORIENTED_EDGE ( 'NONE', *, *, #6767, .F. ) ;
#16594=DIRECTION ( 'NONE',  ( -1.000000000000000000, 1.530638361156006492E-16, 0.000000000000000000 ) ) ;
#16617=FACE_OUTER_BOUND ( 'NONE', #3511, .T. ) ;
#16655=AXIS2_PLACEMENT_3D ( 'NONE', #6943, #18417, #13355 ) ;
#16709=CIRCLE ( 'NONE', #3555, 19.99999999999999289 ) ;
#16717=DIRECTION ( 'NONE',  ( -0.000000000000000000, 1.000000000000000000, -0.000000000000000000 ) ) ;
#16786=AXIS2_PLACEMENT_3D ( 'NONE', #14133, #14016, #3519 ) ;
#16801=DIRECTION ( 'NONE',  ( 1.000000000000000000, -1.084202172485504681E-16, 0.000000000000000000 ) ) ;
#16833=ORIENTED_EDGE ( 'NONE', *, *, #13244, .T. ) ;
#16850=CARTESIAN_POINT ( 'NONE',  ( -34.00000000000000000, -8.251288694035729065, 0.000000000000000000 ) ) ;
#16887=ORIENTED_EDGE ( 'NONE', *, *, #13470, .F. ) ;
#16904=CARTESIAN_POINT ( 'NONE',  ( 17.32050807568884210, -25.00000000000000000, -9.999999999999880984 ) ) ;
#16914=LINE ( 'NONE', #8214, #5064 ) ;
#16933=ORIENTED_EDGE ( 'NONE', *, *, #5165, .T. ) ;
#16956=AXIS2_PLACEMENT_3D ( 'NONE', #10585, #12199, #12419 ) ;
#16980=ORIENTED_EDGE ( 'NONE', *, *, #19282, .T. ) ;
#16981=FACE_OUTER_BOUND ( 'NONE', #17141, .T. ) ;
#16993=DIRECTION ( 'NONE',  ( 1.000000000000000000, 0.000000000000000000, 0.000000000000000000 ) ) ;
#17027=VERTEX_POINT ( 'NONE', #21465 ) ;
#17046=VERTEX_POINT ( 'NONE', #12743 ) ;
#17062=DIRECTION ( 'NONE',  ( 1.296372316667914327E-16, 1.000000000000000000, -0.000000000000000000 ) ) ;
#17064=CARTESIAN_POINT ( 'NONE',  ( 3.877306978638209416E-14, 1.500000000000004885, -12.00000000000000355 ) ) ;
#17079=CIRCLE ( 'NONE', #5029, 3.999999999999998224 ) ;
#17084=DIRECTION ( 'NONE',  ( -1.000000000000000000, 1.264902534566421922E-16, 0.000000000000000000 ) ) ;
#17085=AXIS2_PLACEMENT_3D ( 'NONE', #21074, #20858, #12354 ) ;
#17111=ORIENTED_EDGE ( 'NONE', *, *, #9752, .F. ) ;
#17112=DIRECTION ( 'NONE',  ( 0.9659258262890679791, -0.2588190451025219052, 0.000000000000000000 ) ) ;
#17117=DIRECTION ( 'NONE',  ( -1.000000000000000000, 1.084202172485504681E-16, 0.000000000000000000 ) ) ;
#17141=EDGE_LOOP ( 'NONE', ( #17111, #9155, #1427, #6933 ) ) ;
#17144=CIRCLE ( 'NONE', #316, 4.000000000000145661 ) ;
#17145=PLANE ( 'NONE',  #4704 ) ;
#17208=EDGE_LOOP ( 'NONE', ( #12649, #11412, #17539, #3889, #10111, #8852, #6580, #18747, #6663, #5787, #1658, #229, #3362, #22512, #19939, #11676 ) ) ;
#17211=DIRECTION ( 'NONE',  ( 1.296372316667914327E-16, 1.000000000000000000, -0.000000000000000000 ) ) ;
#17219=CARTESIAN_POINT ( 'NONE',  ( 3.849727973822421485E-15, 1.499999999999997780, 0.000000000000000000 ) ) ;
#17237=ADVANCED_FACE ( 'NONE', ( #20432 ), #18708, .F. ) ;
#17260=VERTEX_POINT ( 'NONE', #3355 ) ;
#17265=DIRECTION ( 'NONE',  ( -1.296372316667914327E-16, -1.000000000000000000, 0.000000000000000000 ) ) ;
#17286=CIRCLE ( 'NONE', #16564, 19.99999999999999289 ) ;
#17291=EDGE_CURVE ( 'NONE', #17046, #5486, #3855, .T. ) ;
#17306=EDGE_LOOP ( 'NONE', ( #3475, #10052, #17557, #8558 ) ) ;
#17330=EDGE_LOOP ( 'NONE', ( #9482, #14255, #19866, #10668 ) ) ;
#17331=FACE_OUTER_BOUND ( 'NONE', #4741, .T. ) ;
#17338=ADVANCED_FACE ( 'NONE', ( #12712 ), #14658, .T. ) ;
#17343=VECTOR ( 'NONE', #16465, 1000.000000000000000 ) ;
#17370=EDGE_CURVE ( 'NONE', #3635, #7032, #9172, .T. ) ;
#17391=AXIS2_PLACEMENT_3D ( 'NONE', #3254, #17211, #1526 ) ;
#17411=CARTESIAN_POINT ( 'NONE',  ( 7.310544252644470693E-15, 28.19616000222403684, 0.000000000000000000 ) ) ;
#17426=CARTESIAN_POINT ( 'NONE',  ( -3.999999999999993339, 28.19616000222403684, 0.000000000000000000 ) ) ;
#17451=CARTESIAN_POINT ( 'NONE',  ( 3.071904583821672593E-15, -4.500000000000010658, 0.000000000000000000 ) ) ;
#17464=CIRCLE ( 'NONE', #5753, 12.00000000000000000 ) ;
#17468=CARTESIAN_POINT ( 'NONE',  ( -17.32050807568840867, -1.500000000000011768, -10.00000000000061284 ) ) ;
#17481=CARTESIAN_POINT ( 'NONE',  ( 19.99999999999999645, -4.500000000000013323, 0.000000000000000000 ) ) ;
#17492=VECTOR ( 'NONE', #19711, 1000.000000000000114 ) ;
#17530=PRODUCT_DEFINITION_FORMATION_WITH_SPECIFIED_SOURCE ( 'ANY', '', #8039, .NOT_KNOWN. ) ;
#17539=ORIENTED_EDGE ( 'NONE', *, *, #9991, .T. ) ;
#17557=ORIENTED_EDGE ( 'NONE', *, *, #4622, .T. ) ;
#17586=ADVANCED_FACE ( 'NONE', ( #1713 ), #21296, .F. ) ;
#17592=DIRECTION ( 'NONE',  ( -1.000000000000000000, 1.275531967630005245E-16, 0.000000000000000000 ) ) ;
#17613=EDGE_CURVE ( 'NONE', #22196, #14743, #20856, .T. ) ;
#17651=EDGE_LOOP ( 'NONE', ( #9187, #16980, #18470, #4831, #10446, #17939, #13530 ) ) ;
#17665=AXIS2_PLACEMENT_3D ( 'NONE', #9993, #4964, #12279 ) ;
#17666=ORIENTED_EDGE ( 'NONE', *, *, #2745, .F. ) ;
#17700=AXIS2_PLACEMENT_3D ( 'NONE', #2376, #12670, #9241 ) ;
#17707=AXIS2_PLACEMENT_3D ( 'NONE', #14878, #6537, #8140 ) ;
#17713=CARTESIAN_POINT ( 'NONE',  ( 13.85640646055118808, -1.500000000000015099, 7.999999999999710454 ) ) ;
#17718=DIRECTION ( 'NONE',  ( 1.296372316667914327E-16, 1.000000000000000000, -0.000000000000000000 ) ) ;
#17738=LINE ( 'NONE', #9034, #22503 ) ;
#17815=ORIENTED_EDGE ( 'NONE', *, *, #4299, .F. ) ;
#17819=AXIS2_PLACEMENT_3D ( 'NONE', #18193, #20035, #2507 ) ;
#17939=ORIENTED_EDGE ( 'NONE', *, *, #9134, .F. ) ;
#17947=PRODUCT_DEFINITION ( 'UNKNOWN', '', #17530, #10949 ) ;
#17966=CARTESIAN_POINT ( 'NONE',  ( 17.32050807568884210, 1.500000000000015099, -9.999999999999880984 ) ) ;
#17980=EDGE_LOOP ( 'NONE', ( #3964, #13572, #2415, #17666 ) ) ;
#17999=ORIENTED_EDGE ( 'NONE', *, *, #10697, .F. ) ;
#18010=DIRECTION ( 'NONE',  ( 1.000000000000000000, -1.275531967630005245E-16, 0.000000000000000000 ) ) ;
#18015=DIRECTION ( 'NONE',  ( -1.296372316667914327E-16, -1.000000000000000000, 0.000000000000000000 ) ) ;
#18022=DIRECTION ( 'NONE',  ( 1.296372316667914327E-16, 1.000000000000000000, -0.000000000000000000 ) ) ;
#18035=EDGE_CURVE ( 'NONE', #9227, #19871, #12772, .T. ) ;
#18041=ORIENTED_EDGE ( 'NONE', *, *, #9991, .F. ) ;
#18044=CIRCLE ( 'NONE', #20978, 4.000000000000145661 ) ;
#18152=CIRCLE ( 'NONE', #577, 12.00000000000000355 ) ;
#18162=DIRECTION ( 'NONE',  ( 1.296372316667914327E-16, 1.000000000000000000, -0.000000000000000000 ) ) ;
#18181=ORIENTED_EDGE ( 'NONE', *, *, #14188, .F. ) ;
#18182=CARTESIAN_POINT ( 'NONE',  ( 10.39230484541330846, -25.00000000000000000, -5.999999999999929834 ) ) ;
#18185=FACE_OUTER_BOUND ( 'NONE', #17208, .T. ) ;
#18193=CARTESIAN_POINT ( 'NONE',  ( 7.310544252644470693E-15, 28.19616000222403684, 0.000000000000000000 ) ) ;
#18204=DIRECTION ( 'NONE',  ( -0.000000000000000000, 1.000000000000000000, -0.000000000000000000 ) ) ;
#18230=CONICAL_SURFACE ( 'NONE', #301, 34.00000000000000000, 1.308996938995746095 ) ;
#18256=ORIENTED_EDGE ( 'NONE', *, *, #10432, .T. ) ;
#18273=AXIS2_PLACEMENT_3D ( 'NONE', #1648, #15491, #16993 ) ;
#18284=CARTESIAN_POINT ( 'NONE',  ( 3.266360431321861887E-15, -2.999999999999995559, 0.000000000000000000 ) ) ;
#18291=CARTESIAN_POINT ( 'NONE',  ( 4.044183821322609990E-15, 3.000000000000006217, 0.000000000000000000 ) ) ;
#18308=VERTEX_POINT ( 'NONE', #6506 ) ;
#18350=EDGE_LOOP ( 'NONE', ( #11137, #34, #11801, #11937 ) ) ;
#18359=ORIENTED_EDGE ( 'NONE', *, *, #1012, .T. ) ;
#18384=ORIENTED_EDGE ( 'NONE', *, *, #17291, .T. ) ;
#18417=DIRECTION ( 'NONE',  ( -1.296372316667914327E-16, -1.000000000000000000, 0.000000000000000000 ) ) ;
#18432=MANIFOLD_SOLID_BREP ( 'Cut-Extrude3', #2377 ) ;
#18457=VERTEX_POINT ( 'NONE', #644 ) ;
#18462=CARTESIAN_POINT ( 'NONE',  ( 19.99999999999999645, -1.500000000000014433, 2.449293598294705724E-15 ) ) ;
#18470=ORIENTED_EDGE ( 'NONE', *, *, #16117, .T. ) ;
#18488=AXIS2_PLACEMENT_3D ( 'NONE', #12026, #13941, #12133 ) ;
#18502=ORIENTED_EDGE ( 'NONE', *, *, #12241, .T. ) ;
#18519=VERTEX_POINT ( 'NONE', #19677 ) ;
#18542=VECTOR ( 'NONE', #10607, 1000.000000000000000 ) ;
#18547=CARTESIAN_POINT ( 'NONE',  ( 4.724946350300523916E-15, 8.251288694035745053, 0.000000000000000000 ) ) ;
#18562=EDGE_CURVE ( 'NONE', #9647, #6470, #3314, .T. ) ;
#18620=AXIS2_PLACEMENT_3D ( 'NONE', #21314, #8937, #5504 ) ;
#18627=DIRECTION ( 'NONE',  ( 1.296372316667914327E-16, 1.000000000000000000, -0.000000000000000000 ) ) ;
#18640=DIRECTION ( 'NONE',  ( -1.000000000000000000, 1.371829164384562918E-16, 0.000000000000000000 ) ) ;
#18678=CARTESIAN_POINT ( 'NONE',  ( 13.85640646055130709, -25.00000000000000000, -4.000000000000099476 ) ) ;
#18699=DIRECTION ( 'NONE',  ( -1.000000000000000000, 1.301042606982605814E-16, 0.000000000000000000 ) ) ;
#18705=ADVANCED_FACE ( 'NONE', ( #21805 ), #21608, .T. ) ;
#18708=CYLINDRICAL_SURFACE ( 'NONE', #22572, 4.000000000000000000 ) ;
#18747=ORIENTED_EDGE ( 'NONE', *, *, #20268, .T. ) ;
#18751=DIRECTION ( 'NONE',  ( 1.296372316667914327E-16, 1.000000000000000000, -0.000000000000000000 ) ) ;
#18770=ORIENTED_EDGE ( 'NONE', *, *, #3565, .F. ) ;
#18827=LINE ( 'NONE', #3363, #21505 ) ;
#18828=ADVANCED_FACE ( 'NONE', ( #1506, #3233 ), #15460, .F. ) ;
#18839=EDGE_LOOP ( 'NONE', ( #1099, #40, #7021, #12530 ) ) ;
#18843=EDGE_CURVE ( 'NONE', #22196, #18519, #13077, .T. ) ;
#18922=DIRECTION ( 'NONE',  ( -1.000000000000000000, 1.084202172485503941E-16, 0.000000000000000000 ) ) ;
#18954=PLANE ( 'NONE',  #14936 ) ;
#18964=ORIENTED_EDGE ( 'NONE', *, *, #5165, .F. ) ;
#19007=FACE_OUTER_BOUND ( 'NONE', #19839, .T. ) ;
#19024=DIRECTION ( 'NONE',  ( 0.000000000000000000, 0.000000000000000000, 1.000000000000000000 ) ) ;
#19058=CYLINDRICAL_SURFACE ( 'NONE', #10352, 19.99999999999999289 ) ;
#19084=CARTESIAN_POINT ( 'NONE',  ( -10.00000000000000000, 1.499999999999997780, 3.000000000000000000 ) ) ;
#19095=DIRECTION ( 'NONE',  ( -1.000000000000000000, 1.371829164384562918E-16, 0.000000000000000000 ) ) ;
#19144=PRODUCT_CONTEXT ( 'NONE', #1399, 'mechanical' ) ;
#19147=CYLINDRICAL_SURFACE ( 'NONE', #1895, 22.12933039895921539 ) ;
#19164=EDGE_CURVE ( 'NONE', #7946, #8065, #18827, .T. ) ;
#19177=EDGE_LOOP ( 'NONE', ( #7715, #15316, #7921, #13319 ) ) ;
#19178=CARTESIAN_POINT ( 'NONE',  ( -10.00000000000000000, -4.824555320336763486, 3.000000000000000000 ) ) ;
#19183=AXIS2_PLACEMENT_3D ( 'NONE', #12440, #17718, #19454 ) ;
#19213=DIRECTION ( 'NONE',  ( 1.296372316667914327E-16, 1.000000000000000000, -0.000000000000000000 ) ) ;
#19247=EDGE_LOOP ( 'NONE', ( #18964, #3616, #1095, #21058 ) ) ;
#19256=CARTESIAN_POINT ( 'NONE',  ( 0.000000000000000000, -1.500000000000015099, 0.000000000000000000 ) ) ;
#19271=DIRECTION ( 'NONE',  ( -1.000000000000000000, 1.296372316667914327E-16, 0.000000000000000000 ) ) ;
#19272=DIRECTION ( 'NONE',  ( -0.000000000000000000, 1.000000000000000000, -0.000000000000000000 ) ) ;
#19277=CYLINDRICAL_SURFACE ( 'NONE', #17819, 22.12933039895921539 ) ;
#19282=EDGE_CURVE ( 'NONE', #19871, #10716, #20070, .T. ) ;
#19288=FACE_BOUND ( 'NONE', #10216, .T. ) ;
#19318=ADVANCED_FACE ( 'NONE', ( #14668 ), #18230, .T. ) ;
#19365=EDGE_CURVE ( 'NONE', #3635, #5980, #14406, .T. ) ;
#19375=CIRCLE ( 'NONE', #21194, 3.999999999999998224 ) ;
#19378=EDGE_CURVE ( 'NONE', #22383, #7, #4230, .T. ) ;
#19420=CARTESIAN_POINT ( 'NONE',  ( 3.071904583821672593E-15, -4.500000000000010658, 0.000000000000000000 ) ) ;
#19454=DIRECTION ( 'NONE',  ( -1.000000000000000000, 1.301042606982605814E-16, 0.000000000000000000 ) ) ;
#19470=DIRECTION ( 'NONE',  ( -1.000000000000000000, 1.084202172485505420E-16, 0.000000000000000000 ) ) ;
#19486=VERTEX_POINT ( 'NONE', #9234 ) ;
#19539=CIRCLE ( 'NONE', #4548, 3.999999999999999112 ) ;
#19556=CARTESIAN_POINT ( 'NONE',  ( -13.85640646055084702, -1.500000000000011768, 7.999999999999705125 ) ) ;
#19568=DIRECTION ( 'NONE',  ( 1.296372316667914327E-16, 1.000000000000000000, -0.000000000000000000 ) ) ;
#19581=PLANE ( 'NONE',  #11884 ) ;
#19625=ORIENTED_EDGE ( 'NONE', *, *, #15805, .T. ) ;
#19635=AXIS2_PLACEMENT_3D ( 'NONE', #3550, #2264, #7538 ) ;
#19650=EDGE_LOOP ( 'NONE', ( #15379, #18256, #5974, #21283 ) ) ;
#19677=CARTESIAN_POINT ( 'NONE',  ( -19.99999999999998934, -4.500000000000007994, 3.306546357697853339E-15 ) ) ;
#19690=FACE_OUTER_BOUND ( 'NONE', #3847, .T. ) ;
#19711=DIRECTION ( 'NONE',  ( -0.9659258262890678681, 0.2588190451025220717, 0.000000000000000000 ) ) ;
#19816=CARTESIAN_POINT ( 'NONE',  ( -33.99999999999998579, 8.251288694035750382, 0.000000000000000000 ) ) ;
#19824=FACE_OUTER_BOUND ( 'NONE', #5506, .T. ) ;
#19839=EDGE_LOOP ( 'NONE', ( #7751, #19625, #20244, #6135 ) ) ;
#19843=ORIENTED_EDGE ( 'NONE', *, *, #18562, .T. ) ;
#19861=CARTESIAN_POINT ( 'NONE',  ( 0.000000000000000000, -25.00000000000000000, 19.99999999999999645 ) ) ;
#19866=ORIENTED_EDGE ( 'NONE', *, *, #10020, .T. ) ;
#19871=VERTEX_POINT ( 'NONE', #8551 ) ;
#19884=CYLINDRICAL_SURFACE ( 'NONE', #5085, 3.999999999999997335 ) ;
#19905=LINE ( 'NONE', #4332, #17343 ) ;
#19916=CIRCLE ( 'NONE', #7466, 3.999999999999998224 ) ;
#19925=CARTESIAN_POINT ( 'NONE',  ( -17.32050807568833051, -25.00000000000000000, -10.00000000000047251 ) ) ;
#19937=DIRECTION ( 'NONE',  ( 1.296372316667914327E-16, 1.000000000000000000, -0.000000000000000000 ) ) ;
#19939=ORIENTED_EDGE ( 'NONE', *, *, #17291, .F. ) ;
#19951=CARTESIAN_POINT ( 'NONE',  ( 2.854018578421813982E-15, -6.180736333215565814, 0.000000000000000000 ) ) ;
#19969=DIRECTION ( 'NONE',  ( -1.000000000000000000, 1.084202172485464991E-16, 0.000000000000000000 ) ) ;
#19975=EDGE_CURVE ( 'NONE', #17260, #6902, #8731, .T. ) ;
#19996=ORIENTED_EDGE ( 'NONE', *, *, #7240, .T. ) ;
#20001=DIRECTION ( 'NONE',  ( -1.000000000000000000, 0.000000000000000000, 0.000000000000000000 ) ) ;
#20028=AXIS2_PLACEMENT_3D ( 'NONE', #2640, #16717, #13251 ) ;
#20035=DIRECTION ( 'NONE',  ( 1.296372316667914327E-16, 1.000000000000000000, -0.000000000000000000 ) ) ;
#20042=VECTOR ( 'NONE', #11136, 1000.000000000000000 ) ;
#20061=LINE ( 'NONE', #18678, #11240 ) ;
#20070=CIRCLE ( 'NONE', #12363, 19.99999999999999289 ) ;
#20130=AXIS2_PLACEMENT_3D ( 'NONE', #4943, #11923, #18922 ) ;
#20142=DIRECTION ( 'NONE',  ( 1.296372316667914327E-16, 1.000000000000000000, -0.000000000000000000 ) ) ;
#20154=FACE_OUTER_BOUND ( 'NONE', #19247, .T. ) ;
#20221=ORIENTED_EDGE ( 'NONE', *, *, #2380, .F. ) ;
#20227=VERTEX_POINT ( 'NONE', #20233 ) ;
#20233=CARTESIAN_POINT ( 'NONE',  ( -11.99999999999999289, 12.49999999999999822, 0.000000000000000000 ) ) ;
#20239=CIRCLE ( 'NONE', #10327, 33.99999999999999289 ) ;
#20244=ORIENTED_EDGE ( 'NONE', *, *, #3317, .T. ) ;
#20268=EDGE_CURVE ( 'NONE', #7946, #9114, #14089, .T. ) ;
#20432=FACE_OUTER_BOUND ( 'NONE', #6103, .T. ) ;
#20458=CARTESIAN_POINT ( 'NONE',  ( 4.044183821322609990E-15, 3.000000000000006217, 0.000000000000000000 ) ) ;
#20503=EDGE_CURVE ( 'NONE', #14743, #15720, #6455, .T. ) ;
#20525=AXIS2_PLACEMENT_3D ( 'NONE', #9226, #517, #21492 ) ;
#20557=ORIENTED_EDGE ( 'NONE', *, *, #15530, .T. ) ;
#20589=FACE_OUTER_BOUND ( 'NONE', #20594, .T. ) ;
#20594=EDGE_LOOP ( 'NONE', ( #8968, #9219, #7864, #4717 ) ) ;
#20658=VECTOR ( 'NONE', #8614, 1000.000000000000227 ) ;
#20665=DIRECTION ( 'NONE',  ( -1.296372316667914327E-16, -1.000000000000000000, 0.000000000000000000 ) ) ;
#20698=FACE_OUTER_BOUND ( 'NONE', #11913, .T. ) ;
#20701=ADVANCED_FACE ( 'NONE', ( #16981 ), #13531, .F. ) ;
#20703=ORIENTED_EDGE ( 'NONE', *, *, #2630, .T. ) ;
#20718=DIRECTION ( 'NONE',  ( -1.000000000000000000, 0.000000000000000000, 0.000000000000000000 ) ) ;
#20741=CARTESIAN_POINT ( 'NONE',  ( -13.85640646055084702, -25.00000000000000000, 7.999999999999705125 ) ) ;
#20786=LINE ( 'NONE', #19178, #12025 ) ;
#20802=DIRECTION ( 'NONE',  ( 1.296372316667914327E-16, 1.000000000000000000, -0.000000000000000000 ) ) ;
#20834=CARTESIAN_POINT ( 'NONE',  ( 17.32050807568869644, -1.500000000000011768, 10.00000000000013323 ) ) ;
#20845=ORIENTED_EDGE ( 'NONE', *, *, #15606, .T. ) ;
#20856=LINE ( 'NONE', #8581, #8244 ) ;
#20858=DIRECTION ( 'NONE',  ( -1.296372316667914327E-16, -1.000000000000000000, 0.000000000000000000 ) ) ;
#20863=CARTESIAN_POINT ( 'NONE',  ( -10.39230484541309174, 1.500000000000008216, 5.999999999999708677 ) ) ;
#20864=EDGE_CURVE ( 'NONE', #10675, #8683, #14314, .T. ) ;
#20871=LINE ( 'NONE', #10081, #12832 ) ;
#20890=LINE ( 'NONE', #8735, #20658 ) ;
#20897=ORIENTED_EDGE ( 'NONE', *, *, #2829, .T. ) ;
#20898=VECTOR ( 'NONE', #7134, 1000.000000000000114 ) ;
#20943=( NAMED_UNIT ( * ) PLANE_ANGLE_UNIT ( ) SI_UNIT ( $, .RADIAN. ) );
#20975=EDGE_LOOP ( 'NONE', ( #5514, #21442, #21449, #16401 ) ) ;
#20978=AXIS2_PLACEMENT_3D ( 'NONE', #21374, #9344, #5671 ) ;
#20981=ORIENTED_EDGE ( 'NONE', *, *, #13765, .F. ) ;
#21022=ORIENTED_EDGE ( 'NONE', *, *, #6271, .T. ) ;
#21058=ORIENTED_EDGE ( 'NONE', *, *, #7240, .F. ) ;
#21073=ORIENTED_EDGE ( 'NONE', *, *, #13793, .T. ) ;
#21074=CARTESIAN_POINT ( 'NONE',  ( 12.00000000000000355, 1.500000000000003553, 0.000000000000000000 ) ) ;
#21078=CONICAL_SURFACE ( 'NONE', #2803, 33.99999999999999289, 1.308996938995745873 ) ;
#21127=CARTESIAN_POINT ( 'NONE',  ( 22.12933039895922249, 28.19616000222403329, 2.710061364035962525E-15 ) ) ;
#21142=AXIS2_PLACEMENT_3D ( 'NONE', #659, #7756, #14956 ) ;
#21178=LINE ( 'NONE', #422, #1373 ) ;
#21194=AXIS2_PLACEMENT_3D ( 'NONE', #5987, #16524, #9541 ) ;
#21199=CARTESIAN_POINT ( 'NONE',  ( 3.460816278822046447E-15, -1.500000000000015099, 0.000000000000000000 ) ) ;
#21227=ADVANCED_FACE ( 'NONE', ( #1595 ), #8583, .F. ) ;
#21247=DIRECTION ( 'NONE',  ( -1.000000000000000000, 1.301042606982605814E-16, 0.000000000000000000 ) ) ;
#21250=FACE_OUTER_BOUND ( 'NONE', #20975, .T. ) ;
#21283=ORIENTED_EDGE ( 'NONE', *, *, #501, .T. ) ;
#21293=FACE_OUTER_BOUND ( 'NONE', #18839, .T. ) ;
#21296=CYLINDRICAL_SURFACE ( 'NONE', #18488, 4.000000000000000000 ) ;
#21314=CARTESIAN_POINT ( 'NONE',  ( 4.724946350300523916E-15, 8.251288694035745053, 0.000000000000000000 ) ) ;
#21336=AXIS2_PLACEMENT_3D ( 'NONE', #494, #21594, #7272 ) ;
#21353=LINE ( 'NONE', #15738, #6817 ) ;
#21374=CARTESIAN_POINT ( 'NONE',  ( -3.418729828831206752E-14, 1.500000000000004885, 15.99999999999970512 ) ) ;
#21381=AXIS2_PLACEMENT_3D ( 'NONE', #5620, #3919, #10889 ) ;
#21384=CARTESIAN_POINT ( 'NONE',  ( 13.85640646055130709, 1.500000000000004885, -8.000000000000097700 ) ) ;
#21392=VERTEX_POINT ( 'NONE', #20834 ) ;
#21400=CARTESIAN_POINT ( 'NONE',  ( 22.12933039895921894, -2.999999999999998668, 2.710061364035962525E-15 ) ) ;
#21408=CARTESIAN_POINT ( 'NONE',  ( 13.85640646055130709, -1.500000000000015099, -8.000000000000097700 ) ) ;
#21420=SHAPE_REPRESENTATION ( 'FLYWHEEL', ( #18273 ), #1444 ) ;
#21435=CIRCLE ( 'NONE', #1684, 4.000000000000000000 ) ;
#21442=ORIENTED_EDGE ( 'NONE', *, *, #21744, .T. ) ;
#21448=ADVANCED_FACE ( 'NONE', ( #19824 ), #11213, .F. ) ;
#21449=ORIENTED_EDGE ( 'NONE', *, *, #22654, .T. ) ;
#21455=DIRECTION ( 'NONE',  ( -1.000000000000000000, 1.275531967630005245E-16, 0.000000000000000000 ) ) ;
#21465=CARTESIAN_POINT ( 'NONE',  ( 12.00000000000000355, 12.49999999999999467, 1.469576158976823947E-15 ) ) ;
#21475=CIRCLE ( 'NONE', #3174, 12.00000000000000000 ) ;
#21491=CARTESIAN_POINT ( 'NONE',  ( 13.85640646055130709, -25.00000000000000000, -8.000000000000097700 ) ) ;
#21492=DIRECTION ( 'NONE',  ( -1.000000000000000000, 1.301042606982605814E-16, 0.000000000000000000 ) ) ;
#21505=VECTOR ( 'NONE', #10321, 1000.000000000000000 ) ;
#21527=AXIS2_PLACEMENT_3D ( 'NONE', #21384, #6963, #12217 ) ;
#21549=CYLINDRICAL_SURFACE ( 'NONE', #6965, 3.999999999999997335 ) ;
#21559=VERTEX_POINT ( 'NONE', #22571 ) ;
#21570=ORIENTED_EDGE ( 'NONE', *, *, #10006, .F. ) ;
#21594=DIRECTION ( 'NONE',  ( 1.296372316667914327E-16, 1.000000000000000000, -0.000000000000000000 ) ) ;
#21608=CONICAL_SURFACE ( 'NONE', #11722, 34.00000000000000000, 1.308996938995746095 ) ;
#21619=CARTESIAN_POINT ( 'NONE',  ( 3.460816278822046447E-15, -1.500000000000011768, 0.000000000000000000 ) ) ;
#21637=ORIENTED_EDGE ( 'NONE', *, *, #9134, .T. ) ;
#21643=DIRECTION ( 'NONE',  ( -0.000000000000000000, -0.000000000000000000, 1.000000000000000000 ) ) ;
#21657=DIRECTION ( 'NONE',  ( -1.000000000000000000, 1.530638361156006492E-16, 0.000000000000000000 ) ) ;
#21664=DIRECTION ( 'NONE',  ( 1.000000000000000000, -1.296372316667914327E-16, 0.000000000000000000 ) ) ;
#21671=DIRECTION ( 'NONE',  ( -1.296372316667914327E-16, -1.000000000000000000, 0.000000000000000000 ) ) ;
#21673=CARTESIAN_POINT ( 'NONE',  ( -33.99999999999999289, 28.19616000222404040, 0.000000000000000000 ) ) ;
#21721=AXIS2_PLACEMENT_3D ( 'NONE', #16441, #7734, #20001 ) ;
#21739=AXIS2_PLACEMENT_3D ( 'NONE', #16481, #15396, #5835 ) ;
#21744=EDGE_CURVE ( 'NONE', #18308, #1985, #21178, .T. ) ;
#21765=DIRECTION ( 'NONE',  ( -1.000000000000000000, 1.530638361156006245E-16, 0.000000000000000000 ) ) ;
#21805=FACE_OUTER_BOUND ( 'NONE', #13580, .T. ) ;
#21806=ADVANCED_FACE ( 'NONE', ( #18185, #881 ), #14840, .F. ) ;
#21855=CARTESIAN_POINT ( 'NONE',  ( 3.849727973822423851E-15, 1.500000000000011768, 0.000000000000000000 ) ) ;
#21883=DIRECTION ( 'NONE',  ( 1.296372316667914327E-16, 1.000000000000000000, -0.000000000000000000 ) ) ;
#21910=AXIS2_PLACEMENT_3D ( 'NONE', #22300, #18627, #6250 ) ;
#21914=ORIENTED_EDGE ( 'NONE', *, *, #17370, .F. ) ;
#21945=ADVANCED_FACE ( 'NONE', ( #20698 ), #10142, .T. ) ;
#21949=VERTEX_POINT ( 'NONE', #9821 ) ;
#21988=ORIENTED_EDGE ( 'NONE', *, *, #4592, .T. ) ;
#21989=EDGE_CURVE ( 'NONE', #2304, #5844, #16914, .T. ) ;
#22012=DIRECTION ( 'NONE',  ( -0.000000000000000000, 1.000000000000000000, -0.000000000000000000 ) ) ;
#22014=CARTESIAN_POINT ( 'NONE',  ( 3.849727973822423851E-15, 1.500000000000011768, 0.000000000000000000 ) ) ;
#22030=DIRECTION ( 'NONE',  ( -1.296372316667914327E-16, -1.000000000000000000, 0.000000000000000000 ) ) ;
#22085=VECTOR ( 'NONE', #6000, 1000.000000000000000 ) ;
#22124=DIRECTION ( 'NONE',  ( -1.000000000000000000, 1.204669080539449590E-16, 0.000000000000000000 ) ) ;
#22147=CARTESIAN_POINT ( 'NONE',  ( 3.877306978638209416E-14, -1.500000000000015099, -12.00000000000000355 ) ) ;
#22187=VECTOR ( 'NONE', #11544, 1000.000000000000000 ) ;
#22196=VERTEX_POINT ( 'NONE', #17481 ) ;
#22218=CARTESIAN_POINT ( 'NONE',  ( 7.310544252644470693E-15, 28.19616000222403684, 0.000000000000000000 ) ) ;
#22300=CARTESIAN_POINT ( 'NONE',  ( 0.000000000000000000, -1.500000000000015099, 0.000000000000000000 ) ) ;
#22355=CARTESIAN_POINT ( 'NONE',  ( 3.849727973822421485E-15, 1.499999999999994449, 0.000000000000000000 ) ) ;
#22383=VERTEX_POINT ( 'NONE', #1276 ) ;
#22398=VERTEX_POINT ( 'NONE', #1735 ) ;
#22408=DIRECTION ( 'NONE',  ( 1.296372316667914327E-16, 1.000000000000000000, -0.000000000000000000 ) ) ;
#22418=EDGE_LOOP ( 'NONE', ( #9573, #21988 ) ) ;
#22422=CARTESIAN_POINT ( 'NONE',  ( -11.99999999999985434, -1.500000000000013767, 0.000000000000000000 ) ) ;
#22427=AXIS2_PLACEMENT_3D ( 'NONE', #3292, #1797, #17592 ) ;
#22428=ORIENTED_EDGE ( 'NONE', *, *, #8209, .F. ) ;
#22503=VECTOR ( 'NONE', #3671, 1000.000000000000000 ) ;
#22512=ORIENTED_EDGE ( 'NONE', *, *, #15091, .T. ) ;
#22545=VECTOR ( 'NONE', #16476, 1000.000000000000000 ) ;
#22565=CARTESIAN_POINT ( 'NONE',  ( 4.000000000000003553, 1.499999999999996447, 0.000000000000000000 ) ) ;
#22571=CARTESIAN_POINT ( 'NONE',  ( -17.32050807568833051, 1.500000000000015099, -10.00000000000047251 ) ) ;
#22572=AXIS2_PLACEMENT_3D ( 'NONE', #5076, #6564, #1398 ) ;
#22579=CARTESIAN_POINT ( 'NONE',  ( 10.39230484541308819, 1.500000000000004885, 6.000000000000008882 ) ) ;
#22634=CARTESIAN_POINT ( 'NONE',  ( 4.456525674222657894E-15, 6.180736333215575584, 0.000000000000000000 ) ) ;
#22654=EDGE_CURVE ( 'NONE', #1985, #7, #15310, .T. ) ;
#22665=EDGE_CURVE ( 'NONE', #5947, #5980, #20786, .T. ) ;
#22672=ADVANCED_FACE ( 'NONE', ( #17331 ), #18954, .F. ) ;
#22691=EDGE_CURVE ( 'NONE', #11067, #5224, #5810, .T. ) ;
#22742=COLOUR_RGB('Off White',0.89,0.88,0.83);
#22743=FILL_AREA_STYLE_COLOUR('',#22742);
#22744=FILL_AREA_STYLE('',(#22743));
#22745=SURFACE_STYLE_FILL_AREA(#22744);
#22746=SURFACE_SIDE_STYLE('',(#22745));
#22747=SURFACE_STYLE_USAGE(.BOTH.,#22746);
#22748=PRESENTATION_STYLE_ASSIGNMENT((#22747));
ENDSEC;
END-ISO-10303-21;
